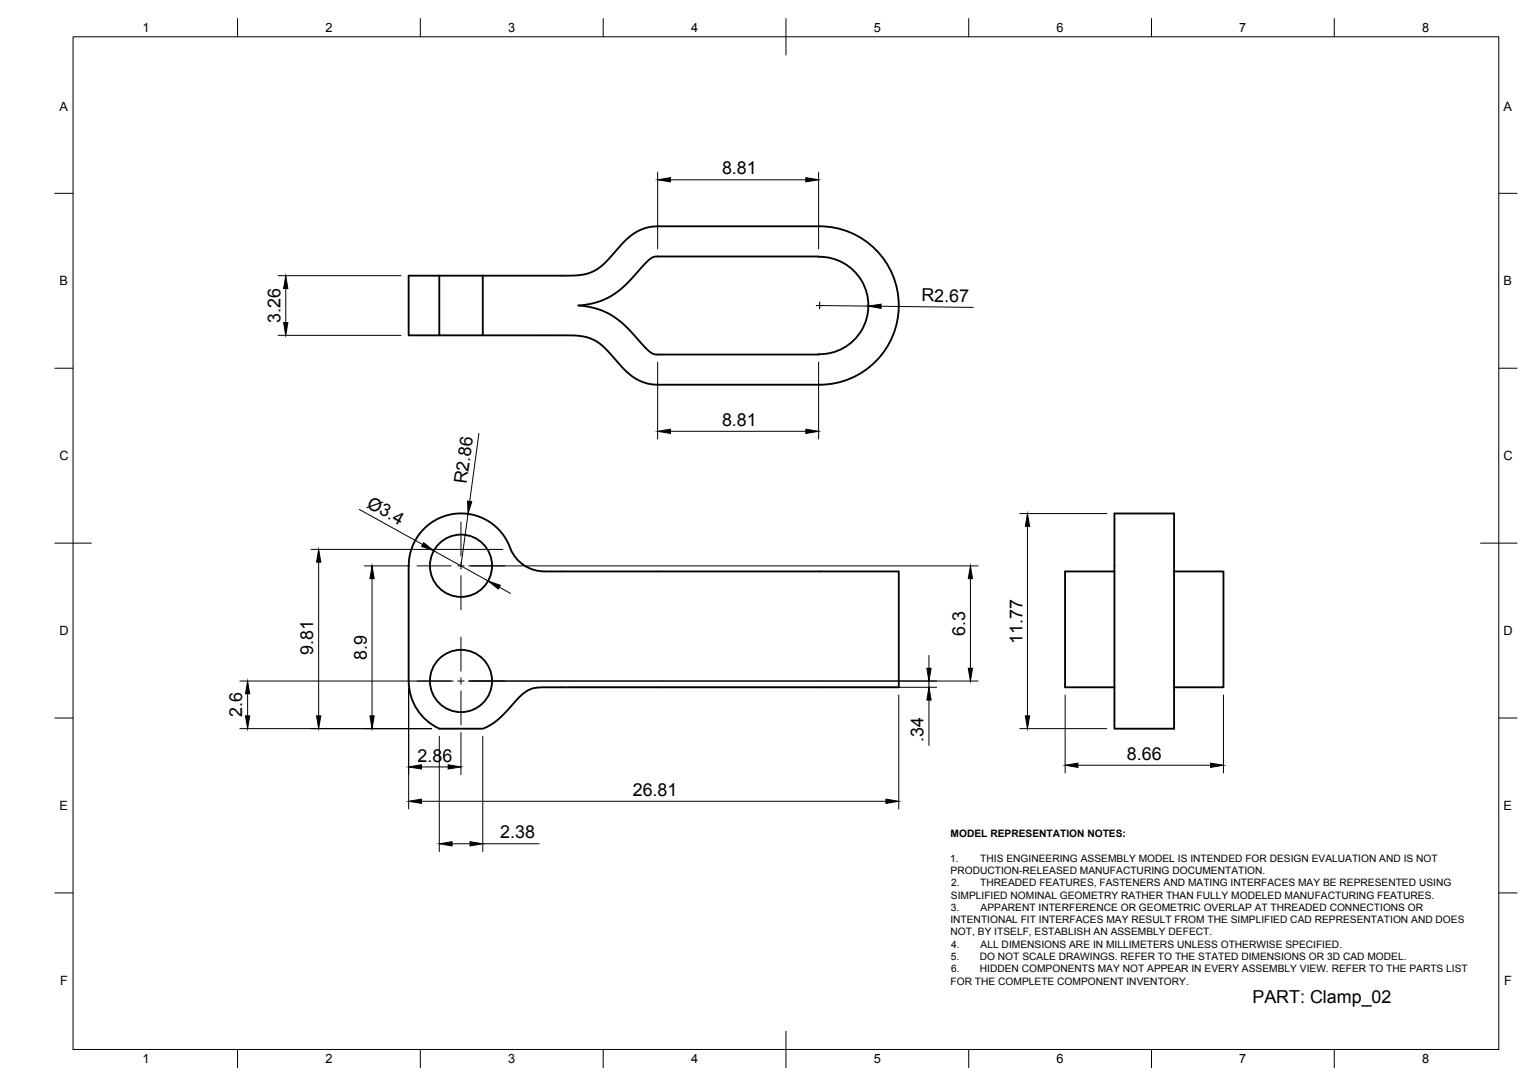
ISO-10303-21;
HEADER;
/* Generated by software containing ST-Developer
 * from STEP Tools, Inc. (www.steptools.com) 
 */

FILE_DESCRIPTION(
/* description */ (''),
/* implementation_level */ '2;1');

FILE_NAME(
/* name */ 'Clamp_02.step',
/* time_stamp */ '2026-10-05T16:20:14-07:00',
/* author */ (''),
/* organization */ (''),
/* preprocessor_version */ 'ST-DEVELOPER v20.2',
/* originating_system */ 'Autodesk Translation Framework v15.15.0.0',
/* authorisation */ '');

FILE_SCHEMA (('AUTOMOTIVE_DESIGN { 1 0 10303 214 3 1 1 }'));
ENDSEC;

DATA;
#10=MECHANICAL_DESIGN_GEOMETRIC_PRESENTATION_REPRESENTATION('',(#254),#23577);
#57=B_SPLINE_SURFACE_WITH_KNOTS('',5,1,((#22213,#22214),(#22215,#22216),
(#22217,#22218),(#22219,#22220),(#22221,#22222),(#22223,#22224),(#22225,
#22226),(#22227,#22228),(#22229,#22230),(#22231,#22232),(#22233,#22234),
(#22235,#22236),(#22237,#22238),(#22239,#22240),(#22241,#22242),(#22243,
#22244),(#22245,#22246),(#22247,#22248),(#22249,#22250),(#22251,#22252)),
 .UNSPECIFIED.,.F.,.F.,.F.,(6,1,1,1,1,1,1,1,1,1,1,1,1,1,1,6),(2,2),(0.,
0.0666666666666667,0.133333333333333,0.2,0.266666666666667,0.333333333333333,
0.4,0.466666666666667,0.533333333333333,0.6,0.666666666666667,0.733333333333333,
0.8,0.866666666666667,0.933333333333333,1.),(0.,1.44),.UNSPECIFIED.);
#58=B_SPLINE_SURFACE_WITH_KNOTS('',3,1,((#22299,#22300),(#22301,#22302),
(#22303,#22304),(#22305,#22306),(#22307,#22308),(#22309,#22310),(#22311,
#22312),(#22313,#22314),(#22315,#22316),(#22317,#22318),(#22319,#22320),
(#22321,#22322),(#22323,#22324),(#22325,#22326),(#22327,#22328),(#22329,
#22330)),.UNSPECIFIED.,.F.,.F.,.F.,(4,3,3,3,3,4),(2,2),(-1.,-0.857074929962035,
-0.680580226328136,-0.49099360586306,-0.247446976985656,0.),(0.,1.44229698166468),
 .UNSPECIFIED.);
#59=B_SPLINE_SURFACE_WITH_KNOTS('',3,1,((#22422,#22423),(#22424,#22425),
(#22426,#22427),(#22428,#22429),(#22430,#22431),(#22432,#22433),(#22434,
#22435),(#22436,#22437),(#22438,#22439),(#22440,#22441),(#22442,#22443),
(#22444,#22445),(#22446,#22447),(#22448,#22449),(#22450,#22451),(#22452,
#22453)),.UNSPECIFIED.,.F.,.F.,.F.,(4,3,3,3,3,4),(2,2),(-1.,-0.857074929962035,
-0.680580226328136,-0.49099360586306,-0.247446976985656,0.),(0.,1.44229698166468),
 .UNSPECIFIED.);
#60=B_SPLINE_SURFACE_WITH_KNOTS('',5,1,((#22519,#22520),(#22521,#22522),
(#22523,#22524),(#22525,#22526),(#22527,#22528),(#22529,#22530),(#22531,
#22532),(#22533,#22534),(#22535,#22536),(#22537,#22538),(#22539,#22540),
(#22541,#22542),(#22543,#22544),(#22545,#22546),(#22547,#22548),(#22549,
#22550),(#22551,#22552),(#22553,#22554),(#22555,#22556),(#22557,#22558)),
 .UNSPECIFIED.,.F.,.F.,.F.,(6,1,1,1,1,1,1,1,1,1,1,1,1,1,1,6),(2,2),(0.,
0.0666666666666667,0.133333333333333,0.2,0.266666666666667,0.333333333333333,
0.4,0.466666666666667,0.533333333333333,0.6,0.666666666666667,0.733333333333333,
0.8,0.866666666666667,0.933333333333333,1.),(0.,2.88),.UNSPECIFIED.);
#61=B_SPLINE_SURFACE_WITH_KNOTS('',5,1,((#22641,#22642),(#22643,#22644),
(#22645,#22646),(#22647,#22648),(#22649,#22650),(#22651,#22652),(#22653,
#22654),(#22655,#22656),(#22657,#22658),(#22659,#22660),(#22661,#22662),
(#22663,#22664),(#22665,#22666),(#22667,#22668),(#22669,#22670),(#22671,
#22672),(#22673,#22674),(#22675,#22676),(#22677,#22678),(#22679,#22680)),
 .UNSPECIFIED.,.F.,.F.,.F.,(6,1,1,1,1,1,1,1,1,1,1,1,1,1,1,6),(2,2),(0.,
0.0666666666666667,0.133333333333333,0.2,0.266666666666667,0.333333333333333,
0.4,0.466666666666667,0.533333333333333,0.6,0.666666666666667,0.733333333333333,
0.8,0.866666666666667,0.933333333333333,1.),(0.,1.44),.UNSPECIFIED.);
#181=B_SPLINE_CURVE_WITH_KNOTS('',5,(#22255,#22256,#22257,#22258,#22259,
#22260,#22261,#22262,#22263,#22264,#22265,#22266,#22267,#22268,#22269,#22270,
#22271,#22272,#22273,#22274),.UNSPECIFIED.,.F.,.F.,(6,1,1,1,1,1,1,1,1,1,
1,1,1,1,1,6),(0.,0.0666666666666667,0.133333333333333,0.2,0.266666666666667,
0.333333333333333,0.4,0.466666666666667,0.533333333333333,0.6,0.666666666666667,
0.733333333333333,0.8,0.866666666666667,0.933333333333333,1.),
 .UNSPECIFIED.);
#182=B_SPLINE_CURVE_WITH_KNOTS('',5,(#22278,#22279,#22280,#22281,#22282,
#22283,#22284,#22285,#22286,#22287,#22288,#22289,#22290,#22291,#22292,#22293,
#22294,#22295,#22296,#22297),.UNSPECIFIED.,.F.,.F.,(6,1,1,1,1,1,1,1,1,1,
1,1,1,1,1,6),(-1.,-0.933333333333333,-0.866666666666667,-0.8,-0.733333333333333,
-0.666666666666667,-0.6,-0.533333333333333,-0.466666666666667,-0.4,-0.333333333333333,
-0.266666666666667,-0.2,-0.133333333333333,-0.0666666666666667,0.),
 .UNSPECIFIED.);
#183=B_SPLINE_CURVE_WITH_KNOTS('',3,(#22335,#22336,#22337,#22338,#22339,
#22340,#22341,#22342,#22343,#22344,#22345,#22346,#22347,#22348,#22349,#22350),
 .UNSPECIFIED.,.F.,.F.,(4,3,3,3,3,4),(0.,0.247446976985656,0.49099360586306,
0.680580226328136,0.857074929962035,0.858875452739877),.UNSPECIFIED.);
#184=B_SPLINE_CURVE_WITH_KNOTS('',3,(#22353,#22354,#22355,#22356,#22357,
#22358,#22359,#22360,#22361,#22362,#22363,#22364),.UNSPECIFIED.,.F.,.F.,
(4,2,2,2,2,4),(-0.363889062449988,-0.363126279310584,-0.288348844096792,
-0.208024613752543,-0.10483855837836,0.),.UNSPECIFIED.);
#185=B_SPLINE_CURVE_WITH_KNOTS('',5,(#22372,#22373,#22374,#22375,#22376,
#22377,#22378,#22379,#22380,#22381,#22382,#22383,#22384,#22385,#22386,#22387,
#22388,#22389,#22390,#22391),.UNSPECIFIED.,.F.,.F.,(6,1,1,1,1,1,1,1,1,1,
1,1,1,1,1,6),(0.,0.0666666666666667,0.133333333333333,0.2,0.266666666666667,
0.333333333333333,0.4,0.466666666666667,0.533333333333333,0.6,0.666666666666667,
0.733333333333333,0.8,0.866666666666667,0.933333333333333,0.989745839682859),
 .UNSPECIFIED.);
#186=B_SPLINE_CURVE_WITH_KNOTS('',3,(#22455,#22456,#22457,#22458,#22459,
#22460,#22461,#22462,#22463,#22464,#22465,#22466),.UNSPECIFIED.,.F.,.F.,
(4,2,2,2,2,4),(-0.363889062449988,-0.363126279310585,-0.288348844096793,
-0.208024613752544,-0.10483855837836,0.),.UNSPECIFIED.);
#187=B_SPLINE_CURVE_WITH_KNOTS('',3,(#22469,#22470,#22471,#22472,#22473,
#22474,#22475,#22476,#22477,#22478,#22479,#22480,#22481,#22482,#22483,#22484),
 .UNSPECIFIED.,.F.,.F.,(4,3,3,3,3,4),(0.,0.247446976985656,0.49099360586306,
0.680580226328136,0.857074929962035,0.858875452739877),.UNSPECIFIED.);
#188=B_SPLINE_CURVE_WITH_KNOTS('',5,(#22491,#22492,#22493,#22494,#22495,
#22496,#22497,#22498,#22499,#22500,#22501,#22502,#22503,#22504,#22505,#22506,
#22507,#22508,#22509,#22510),.UNSPECIFIED.,.F.,.F.,(6,1,1,1,1,1,1,1,1,1,
1,1,1,1,1,6),(0.,0.0666666666666667,0.133333333333333,0.2,0.266666666666667,
0.333333333333333,0.4,0.466666666666667,0.533333333333333,0.6,0.666666666666667,
0.733333333333333,0.8,0.866666666666667,0.933333333333333,1.),
 .UNSPECIFIED.);
#189=B_SPLINE_CURVE_WITH_KNOTS('',5,(#22561,#22562,#22563,#22564,#22565,
#22566,#22567,#22568,#22569,#22570,#22571,#22572,#22573,#22574,#22575,#22576,
#22577,#22578,#22579,#22580),.UNSPECIFIED.,.F.,.F.,(6,1,1,1,1,1,1,1,1,1,
1,1,1,1,1,6),(0.,0.0666666666666667,0.133333333333333,0.2,0.266666666666667,
0.333333333333333,0.4,0.466666666666667,0.533333333333333,0.6,0.666666666666667,
0.733333333333333,0.8,0.866666666666667,0.933333333333333,0.989745839682859),
 .UNSPECIFIED.);
#190=B_SPLINE_CURVE_WITH_KNOTS('',5,(#22605,#22606,#22607,#22608,#22609,
#22610,#22611,#22612,#22613,#22614,#22615,#22616,#22617,#22618,#22619,#22620,
#22621,#22622,#22623,#22624),.UNSPECIFIED.,.F.,.F.,(6,1,1,1,1,1,1,1,1,1,
1,1,1,1,1,6),(-1.,-0.933333333333333,-0.866666666666667,-0.8,-0.733333333333333,
-0.666666666666667,-0.6,-0.533333333333333,-0.466666666666667,-0.4,-0.333333333333333,
-0.266666666666667,-0.2,-0.133333333333333,-0.0666666666666667,0.),
 .UNSPECIFIED.);
#236=SHAPE_REPRESENTATION_RELATIONSHIP('SRR','None',#23619,#245);
#245=ADVANCED_BREP_SHAPE_REPRESENTATION('',(#263),#23575);
#254=STYLED_ITEM('',(#23666),#263);
#263=MANIFOLD_SOLID_BREP('Body1',#4164);
#294=FACE_BOUND('',#822,.T.);
#295=FACE_BOUND('',#823,.T.);
#296=FACE_BOUND('',#829,.T.);
#297=FACE_BOUND('',#836,.T.);
#298=FACE_BOUND('',#842,.T.);
#299=FACE_BOUND('',#843,.T.);
#377=PLANE('',#4574);
#378=PLANE('',#4580);
#379=PLANE('',#4581);
#380=PLANE('',#4582);
#381=PLANE('',#4583);
#382=PLANE('',#4586);
#383=PLANE('',#4593);
#384=PLANE('',#4600);
#385=PLANE('',#4601);
#386=PLANE('',#4602);
#387=PLANE('',#4605);
#388=PLANE('',#4606);
#564=FACE_OUTER_BOUND('',#819,.T.);
#565=FACE_OUTER_BOUND('',#820,.T.);
#566=FACE_OUTER_BOUND('',#821,.T.);
#567=FACE_OUTER_BOUND('',#824,.T.);
#568=FACE_OUTER_BOUND('',#825,.T.);
#569=FACE_OUTER_BOUND('',#826,.T.);
#570=FACE_OUTER_BOUND('',#827,.T.);
#571=FACE_OUTER_BOUND('',#828,.T.);
#572=FACE_OUTER_BOUND('',#830,.T.);
#573=FACE_OUTER_BOUND('',#831,.T.);
#574=FACE_OUTER_BOUND('',#832,.T.);
#575=FACE_OUTER_BOUND('',#833,.T.);
#576=FACE_OUTER_BOUND('',#834,.T.);
#577=FACE_OUTER_BOUND('',#835,.T.);
#578=FACE_OUTER_BOUND('',#837,.T.);
#579=FACE_OUTER_BOUND('',#838,.T.);
#580=FACE_OUTER_BOUND('',#839,.T.);
#581=FACE_OUTER_BOUND('',#840,.T.);
#582=FACE_OUTER_BOUND('',#841,.T.);
#583=FACE_OUTER_BOUND('',#844,.T.);
#584=FACE_OUTER_BOUND('',#845,.T.);
#585=FACE_OUTER_BOUND('',#846,.T.);
#586=FACE_OUTER_BOUND('',#847,.T.);
#587=FACE_OUTER_BOUND('',#848,.T.);
#819=EDGE_LOOP('',(#3565,#3566,#3567,#3568));
#820=EDGE_LOOP('',(#3569,#3570,#3571,#3572));
#821=EDGE_LOOP('',(#3573,#3574,#3575,#3576,#3577,#3578,#3579,#3580,#3581));
#822=EDGE_LOOP('',(#3582));
#823=EDGE_LOOP('',(#3583));
#824=EDGE_LOOP('',(#3584,#3585,#3586,#3587));
#825=EDGE_LOOP('',(#3588,#3589,#3590,#3591));
#826=EDGE_LOOP('',(#3592,#3593,#3594,#3595));
#827=EDGE_LOOP('',(#3596,#3597,#3598,#3599));
#828=EDGE_LOOP('',(#3600,#3601,#3602,#3603,#3604,#3605,#3606,#3607));
#829=EDGE_LOOP('',(#3608,#3609,#3610,#3611,#3612,#3613,#3614));
#830=EDGE_LOOP('',(#3615,#3616,#3617,#3618));
#831=EDGE_LOOP('',(#3619,#3620,#3621,#3622));
#832=EDGE_LOOP('',(#3623,#3624,#3625,#3626));
#833=EDGE_LOOP('',(#3627,#3628,#3629,#3630));
#834=EDGE_LOOP('',(#3631,#3632,#3633,#3634));
#835=EDGE_LOOP('',(#3635,#3636,#3637,#3638,#3639,#3640,#3641,#3642));
#836=EDGE_LOOP('',(#3643,#3644,#3645,#3646,#3647,#3648,#3649));
#837=EDGE_LOOP('',(#3650,#3651,#3652,#3653));
#838=EDGE_LOOP('',(#3654,#3655,#3656,#3657));
#839=EDGE_LOOP('',(#3658,#3659,#3660,#3661));
#840=EDGE_LOOP('',(#3662,#3663,#3664,#3665));
#841=EDGE_LOOP('',(#3666,#3667,#3668,#3669,#3670,#3671,#3672,#3673,#3674));
#842=EDGE_LOOP('',(#3675));
#843=EDGE_LOOP('',(#3676));
#844=EDGE_LOOP('',(#3677,#3678,#3679,#3680));
#845=EDGE_LOOP('',(#3681,#3682,#3683,#3684));
#846=EDGE_LOOP('',(#3685,#3686,#3687,#3688));
#847=EDGE_LOOP('',(#3689,#3690,#3691,#3692));
#848=EDGE_LOOP('',(#3693,#3694,#3695,#3696));
#1102=LINE('',#22276,#1387);
#1103=LINE('',#22298,#1388);
#1104=LINE('',#22333,#1389);
#1105=LINE('',#22352,#1390);
#1106=LINE('',#22370,#1391);
#1107=LINE('',#22392,#1392);
#1108=LINE('',#22394,#1393);
#1109=LINE('',#22399,#1394);
#1110=LINE('',#22406,#1395);
#1111=LINE('',#22408,#1396);
#1112=LINE('',#22409,#1397);
#1113=LINE('',#22413,#1398);
#1114=LINE('',#22415,#1399);
#1115=LINE('',#22417,#1400);
#1116=LINE('',#22418,#1401);
#1117=LINE('',#22420,#1402);
#1118=LINE('',#22421,#1403);
#1119=LINE('',#22468,#1404);
#1120=LINE('',#22487,#1405);
#1121=LINE('',#22489,#1406);
#1122=LINE('',#22512,#1407);
#1123=LINE('',#22517,#1408);
#1124=LINE('',#22518,#1409);
#1125=LINE('',#22560,#1410);
#1126=LINE('',#22583,#1411);
#1127=LINE('',#22584,#1412);
#1128=LINE('',#22587,#1413);
#1129=LINE('',#22591,#1414);
#1130=LINE('',#22594,#1415);
#1131=LINE('',#22597,#1416);
#1132=LINE('',#22603,#1417);
#1133=LINE('',#22625,#1418);
#1134=LINE('',#22627,#1419);
#1135=LINE('',#22629,#1420);
#1136=LINE('',#22634,#1421);
#1137=LINE('',#22638,#1422);
#1138=LINE('',#22640,#1423);
#1139=LINE('',#22681,#1424);
#1140=LINE('',#22682,#1425);
#1141=LINE('',#22685,#1426);
#1142=LINE('',#22688,#1427);
#1143=LINE('',#22690,#1428);
#1387=VECTOR('',#5509,10.);
#1388=VECTOR('',#5510,10.);
#1389=VECTOR('',#5511,10.);
#1390=VECTOR('',#5512,10.);
#1391=VECTOR('',#5517,10.);
#1392=VECTOR('',#5518,10.);
#1393=VECTOR('',#5519,10.);
#1394=VECTOR('',#5524,10.);
#1395=VECTOR('',#5531,10.);
#1396=VECTOR('',#5532,10.);
#1397=VECTOR('',#5533,10.);
#1398=VECTOR('',#5536,10.);
#1399=VECTOR('',#5537,10.);
#1400=VECTOR('',#5538,10.);
#1401=VECTOR('',#5539,10.);
#1402=VECTOR('',#5542,10.);
#1403=VECTOR('',#5543,10.);
#1404=VECTOR('',#5544,10.);
#1405=VECTOR('',#5547,10.);
#1406=VECTOR('',#5548,10.);
#1407=VECTOR('',#5549,10.);
#1408=VECTOR('',#5554,10.);
#1409=VECTOR('',#5555,10.);
#1410=VECTOR('',#5556,10.);
#1411=VECTOR('',#5559,10.);
#1412=VECTOR('',#5560,10.);
#1413=VECTOR('',#5563,10.);
#1414=VECTOR('',#5568,10.);
#1415=VECTOR('',#5571,10.);
#1416=VECTOR('',#5574,10.);
#1417=VECTOR('',#5581,10.);
#1418=VECTOR('',#5582,10.);
#1419=VECTOR('',#5583,10.);
#1420=VECTOR('',#5584,10.);
#1421=VECTOR('',#5591,1.70133516896762);
#1422=VECTOR('',#5596,1.70133516896762);
#1423=VECTOR('',#5599,10.);
#1424=VECTOR('',#5600,10.);
#1425=VECTOR('',#5601,10.);
#1426=VECTOR('',#5606,10.);
#1427=VECTOR('',#5611,10.);
#1428=VECTOR('',#5614,10.);
#1584=CIRCLE('',#4575,2.8615696413584);
#1585=CIRCLE('',#4576,1.99589528357813);
#1586=CIRCLE('',#4577,2.8615696413584);
#1587=CIRCLE('',#4578,1.70133516896762);
#1588=CIRCLE('',#4579,1.70133516896762);
#1589=CIRCLE('',#4584,4.33051922028271);
#1590=CIRCLE('',#4585,2.66551922028271);
#1591=CIRCLE('',#4588,2.8615696413584);
#1592=CIRCLE('',#4590,2.8615696413584);
#1593=CIRCLE('',#4592,1.99589528357813);
#1594=CIRCLE('',#4594,4.33051922028271);
#1595=CIRCLE('',#4595,2.66551922028271);
#1596=CIRCLE('',#4597,1.70133516896762);
#1597=CIRCLE('',#4599,1.70133516896762);
#1951=VERTEX_POINT('',#22253);
#1952=VERTEX_POINT('',#22254);
#1953=VERTEX_POINT('',#22275);
#1954=VERTEX_POINT('',#22277);
#1955=VERTEX_POINT('',#22331);
#1956=VERTEX_POINT('',#22332);
#1957=VERTEX_POINT('',#22334);
#1958=VERTEX_POINT('',#22351);
#1959=VERTEX_POINT('',#22366);
#1960=VERTEX_POINT('',#22367);
#1961=VERTEX_POINT('',#22369);
#1962=VERTEX_POINT('',#22371);
#1963=VERTEX_POINT('',#22393);
#1964=VERTEX_POINT('',#22395);
#1965=VERTEX_POINT('',#22397);
#1966=VERTEX_POINT('',#22400);
#1967=VERTEX_POINT('',#22402);
#1968=VERTEX_POINT('',#22405);
#1969=VERTEX_POINT('',#22407);
#1970=VERTEX_POINT('',#22411);
#1971=VERTEX_POINT('',#22412);
#1972=VERTEX_POINT('',#22414);
#1973=VERTEX_POINT('',#22416);
#1974=VERTEX_POINT('',#22454);
#1975=VERTEX_POINT('',#22467);
#1976=VERTEX_POINT('',#22486);
#1977=VERTEX_POINT('',#22488);
#1978=VERTEX_POINT('',#22490);
#1979=VERTEX_POINT('',#22511);
#1980=VERTEX_POINT('',#22514);
#1981=VERTEX_POINT('',#22516);
#1982=VERTEX_POINT('',#22559);
#1983=VERTEX_POINT('',#22582);
#1984=VERTEX_POINT('',#22586);
#1985=VERTEX_POINT('',#22590);
#1986=VERTEX_POINT('',#22592);
#1987=VERTEX_POINT('',#22596);
#1988=VERTEX_POINT('',#22600);
#1989=VERTEX_POINT('',#22602);
#1990=VERTEX_POINT('',#22604);
#1991=VERTEX_POINT('',#22626);
#1992=VERTEX_POINT('',#22628);
#1993=VERTEX_POINT('',#22632);
#1994=VERTEX_POINT('',#22636);
#2499=EDGE_CURVE('',#1951,#1952,#181,.T.);
#2500=EDGE_CURVE('',#1951,#1953,#1102,.T.);
#2501=EDGE_CURVE('',#1954,#1953,#182,.T.);
#2502=EDGE_CURVE('',#1952,#1954,#1103,.T.);
#2503=EDGE_CURVE('',#1955,#1956,#1104,.T.);
#2504=EDGE_CURVE('',#1957,#1955,#183,.T.);
#2505=EDGE_CURVE('',#1957,#1958,#1105,.T.);
#2506=EDGE_CURVE('',#1956,#1958,#184,.T.);
#2507=EDGE_CURVE('',#1959,#1960,#1584,.T.);
#2508=EDGE_CURVE('',#1959,#1961,#1106,.T.);
#2509=EDGE_CURVE('',#1962,#1961,#185,.T.);
#2510=EDGE_CURVE('',#1952,#1962,#1107,.T.);
#2511=EDGE_CURVE('',#1963,#1954,#1108,.T.);
#2512=EDGE_CURVE('',#1964,#1963,#1585,.T.);
#2513=EDGE_CURVE('',#1965,#1964,#1586,.T.);
#2514=EDGE_CURVE('',#1960,#1965,#1109,.T.);
#2515=EDGE_CURVE('',#1966,#1966,#1587,.T.);
#2516=EDGE_CURVE('',#1967,#1967,#1588,.T.);
#2517=EDGE_CURVE('',#1968,#1951,#1110,.T.);
#2518=EDGE_CURVE('',#1968,#1969,#1111,.T.);
#2519=EDGE_CURVE('',#1953,#1969,#1112,.T.);
#2520=EDGE_CURVE('',#1970,#1971,#1113,.T.);
#2521=EDGE_CURVE('',#1970,#1972,#1114,.T.);
#2522=EDGE_CURVE('',#1973,#1972,#1115,.T.);
#2523=EDGE_CURVE('',#1971,#1973,#1116,.T.);
#2524=EDGE_CURVE('',#1958,#1970,#1117,.T.);
#2525=EDGE_CURVE('',#1972,#1957,#1118,.T.);
#2526=EDGE_CURVE('',#1956,#1974,#186,.T.);
#2527=EDGE_CURVE('',#1975,#1974,#1119,.T.);
#2528=EDGE_CURVE('',#1975,#1955,#187,.T.);
#2529=EDGE_CURVE('',#1962,#1976,#1120,.T.);
#2530=EDGE_CURVE('',#1977,#1976,#1121,.T.);
#2531=EDGE_CURVE('',#1978,#1977,#188,.T.);
#2532=EDGE_CURVE('',#1979,#1978,#1122,.T.);
#2533=EDGE_CURVE('',#1968,#1979,#1589,.T.);
#2534=EDGE_CURVE('',#1971,#1980,#1590,.T.);
#2535=EDGE_CURVE('',#1981,#1980,#1123,.T.);
#2536=EDGE_CURVE('',#1974,#1981,#1124,.T.);
#2537=EDGE_CURVE('',#1982,#1961,#1125,.T.);
#2538=EDGE_CURVE('',#1976,#1982,#189,.T.);
#2539=EDGE_CURVE('',#1959,#1983,#1126,.T.);
#2540=EDGE_CURVE('',#1983,#1982,#1127,.T.);
#2541=EDGE_CURVE('',#1984,#1960,#1128,.T.);
#2542=EDGE_CURVE('',#1983,#1984,#1591,.T.);
#2543=EDGE_CURVE('',#1964,#1985,#1129,.T.);
#2544=EDGE_CURVE('',#1986,#1985,#1592,.T.);
#2545=EDGE_CURVE('',#1965,#1986,#1130,.T.);
#2546=EDGE_CURVE('',#1963,#1987,#1131,.T.);
#2547=EDGE_CURVE('',#1985,#1987,#1593,.T.);
#2548=EDGE_CURVE('',#1988,#1969,#1594,.T.);
#2549=EDGE_CURVE('',#1989,#1988,#1132,.T.);
#2550=EDGE_CURVE('',#1990,#1989,#190,.T.);
#2551=EDGE_CURVE('',#1987,#1990,#1133,.T.);
#2552=EDGE_CURVE('',#1991,#1975,#1134,.T.);
#2553=EDGE_CURVE('',#1992,#1991,#1135,.T.);
#2554=EDGE_CURVE('',#1992,#1973,#1595,.T.);
#2555=EDGE_CURVE('',#1993,#1993,#1596,.T.);
#2556=EDGE_CURVE('',#1993,#1966,#1136,.T.);
#2557=EDGE_CURVE('',#1994,#1994,#1597,.T.);
#2558=EDGE_CURVE('',#1994,#1967,#1137,.T.);
#2559=EDGE_CURVE('',#1984,#1986,#1138,.T.);
#2560=EDGE_CURVE('',#1977,#1990,#1139,.T.);
#2561=EDGE_CURVE('',#1978,#1989,#1140,.T.);
#2562=EDGE_CURVE('',#1979,#1988,#1141,.T.);
#2563=EDGE_CURVE('',#1980,#1992,#1142,.T.);
#2564=EDGE_CURVE('',#1981,#1991,#1143,.T.);
#3565=ORIENTED_EDGE('',*,*,#2499,.F.);
#3566=ORIENTED_EDGE('',*,*,#2500,.T.);
#3567=ORIENTED_EDGE('',*,*,#2501,.F.);
#3568=ORIENTED_EDGE('',*,*,#2502,.F.);
#3569=ORIENTED_EDGE('',*,*,#2503,.F.);
#3570=ORIENTED_EDGE('',*,*,#2504,.F.);
#3571=ORIENTED_EDGE('',*,*,#2505,.T.);
#3572=ORIENTED_EDGE('',*,*,#2506,.F.);
#3573=ORIENTED_EDGE('',*,*,#2507,.F.);
#3574=ORIENTED_EDGE('',*,*,#2508,.T.);
#3575=ORIENTED_EDGE('',*,*,#2509,.F.);
#3576=ORIENTED_EDGE('',*,*,#2510,.F.);
#3577=ORIENTED_EDGE('',*,*,#2502,.T.);
#3578=ORIENTED_EDGE('',*,*,#2511,.F.);
#3579=ORIENTED_EDGE('',*,*,#2512,.F.);
#3580=ORIENTED_EDGE('',*,*,#2513,.F.);
#3581=ORIENTED_EDGE('',*,*,#2514,.F.);
#3582=ORIENTED_EDGE('',*,*,#2515,.F.);
#3583=ORIENTED_EDGE('',*,*,#2516,.F.);
#3584=ORIENTED_EDGE('',*,*,#2517,.F.);
#3585=ORIENTED_EDGE('',*,*,#2518,.T.);
#3586=ORIENTED_EDGE('',*,*,#2519,.F.);
#3587=ORIENTED_EDGE('',*,*,#2500,.F.);
#3588=ORIENTED_EDGE('',*,*,#2520,.F.);
#3589=ORIENTED_EDGE('',*,*,#2521,.T.);
#3590=ORIENTED_EDGE('',*,*,#2522,.F.);
#3591=ORIENTED_EDGE('',*,*,#2523,.F.);
#3592=ORIENTED_EDGE('',*,*,#2524,.F.);
#3593=ORIENTED_EDGE('',*,*,#2505,.F.);
#3594=ORIENTED_EDGE('',*,*,#2525,.F.);
#3595=ORIENTED_EDGE('',*,*,#2521,.F.);
#3596=ORIENTED_EDGE('',*,*,#2503,.T.);
#3597=ORIENTED_EDGE('',*,*,#2526,.T.);
#3598=ORIENTED_EDGE('',*,*,#2527,.F.);
#3599=ORIENTED_EDGE('',*,*,#2528,.T.);
#3600=ORIENTED_EDGE('',*,*,#2529,.T.);
#3601=ORIENTED_EDGE('',*,*,#2530,.F.);
#3602=ORIENTED_EDGE('',*,*,#2531,.F.);
#3603=ORIENTED_EDGE('',*,*,#2532,.F.);
#3604=ORIENTED_EDGE('',*,*,#2533,.F.);
#3605=ORIENTED_EDGE('',*,*,#2517,.T.);
#3606=ORIENTED_EDGE('',*,*,#2499,.T.);
#3607=ORIENTED_EDGE('',*,*,#2510,.T.);
#3608=ORIENTED_EDGE('',*,*,#2506,.T.);
#3609=ORIENTED_EDGE('',*,*,#2524,.T.);
#3610=ORIENTED_EDGE('',*,*,#2520,.T.);
#3611=ORIENTED_EDGE('',*,*,#2534,.T.);
#3612=ORIENTED_EDGE('',*,*,#2535,.F.);
#3613=ORIENTED_EDGE('',*,*,#2536,.F.);
#3614=ORIENTED_EDGE('',*,*,#2526,.F.);
#3615=ORIENTED_EDGE('',*,*,#2537,.F.);
#3616=ORIENTED_EDGE('',*,*,#2538,.F.);
#3617=ORIENTED_EDGE('',*,*,#2529,.F.);
#3618=ORIENTED_EDGE('',*,*,#2509,.T.);
#3619=ORIENTED_EDGE('',*,*,#2539,.T.);
#3620=ORIENTED_EDGE('',*,*,#2540,.T.);
#3621=ORIENTED_EDGE('',*,*,#2537,.T.);
#3622=ORIENTED_EDGE('',*,*,#2508,.F.);
#3623=ORIENTED_EDGE('',*,*,#2541,.F.);
#3624=ORIENTED_EDGE('',*,*,#2542,.F.);
#3625=ORIENTED_EDGE('',*,*,#2539,.F.);
#3626=ORIENTED_EDGE('',*,*,#2507,.T.);
#3627=ORIENTED_EDGE('',*,*,#2543,.T.);
#3628=ORIENTED_EDGE('',*,*,#2544,.F.);
#3629=ORIENTED_EDGE('',*,*,#2545,.F.);
#3630=ORIENTED_EDGE('',*,*,#2513,.T.);
#3631=ORIENTED_EDGE('',*,*,#2546,.T.);
#3632=ORIENTED_EDGE('',*,*,#2547,.F.);
#3633=ORIENTED_EDGE('',*,*,#2543,.F.);
#3634=ORIENTED_EDGE('',*,*,#2512,.T.);
#3635=ORIENTED_EDGE('',*,*,#2546,.F.);
#3636=ORIENTED_EDGE('',*,*,#2511,.T.);
#3637=ORIENTED_EDGE('',*,*,#2501,.T.);
#3638=ORIENTED_EDGE('',*,*,#2519,.T.);
#3639=ORIENTED_EDGE('',*,*,#2548,.F.);
#3640=ORIENTED_EDGE('',*,*,#2549,.F.);
#3641=ORIENTED_EDGE('',*,*,#2550,.F.);
#3642=ORIENTED_EDGE('',*,*,#2551,.F.);
#3643=ORIENTED_EDGE('',*,*,#2528,.F.);
#3644=ORIENTED_EDGE('',*,*,#2552,.F.);
#3645=ORIENTED_EDGE('',*,*,#2553,.F.);
#3646=ORIENTED_EDGE('',*,*,#2554,.T.);
#3647=ORIENTED_EDGE('',*,*,#2522,.T.);
#3648=ORIENTED_EDGE('',*,*,#2525,.T.);
#3649=ORIENTED_EDGE('',*,*,#2504,.T.);
#3650=ORIENTED_EDGE('',*,*,#2555,.F.);
#3651=ORIENTED_EDGE('',*,*,#2556,.T.);
#3652=ORIENTED_EDGE('',*,*,#2515,.T.);
#3653=ORIENTED_EDGE('',*,*,#2556,.F.);
#3654=ORIENTED_EDGE('',*,*,#2557,.F.);
#3655=ORIENTED_EDGE('',*,*,#2558,.T.);
#3656=ORIENTED_EDGE('',*,*,#2516,.T.);
#3657=ORIENTED_EDGE('',*,*,#2558,.F.);
#3658=ORIENTED_EDGE('',*,*,#2545,.T.);
#3659=ORIENTED_EDGE('',*,*,#2559,.F.);
#3660=ORIENTED_EDGE('',*,*,#2541,.T.);
#3661=ORIENTED_EDGE('',*,*,#2514,.T.);
#3662=ORIENTED_EDGE('',*,*,#2531,.T.);
#3663=ORIENTED_EDGE('',*,*,#2560,.T.);
#3664=ORIENTED_EDGE('',*,*,#2550,.T.);
#3665=ORIENTED_EDGE('',*,*,#2561,.F.);
#3666=ORIENTED_EDGE('',*,*,#2542,.T.);
#3667=ORIENTED_EDGE('',*,*,#2559,.T.);
#3668=ORIENTED_EDGE('',*,*,#2544,.T.);
#3669=ORIENTED_EDGE('',*,*,#2547,.T.);
#3670=ORIENTED_EDGE('',*,*,#2551,.T.);
#3671=ORIENTED_EDGE('',*,*,#2560,.F.);
#3672=ORIENTED_EDGE('',*,*,#2530,.T.);
#3673=ORIENTED_EDGE('',*,*,#2538,.T.);
#3674=ORIENTED_EDGE('',*,*,#2540,.F.);
#3675=ORIENTED_EDGE('',*,*,#2555,.T.);
#3676=ORIENTED_EDGE('',*,*,#2557,.T.);
#3677=ORIENTED_EDGE('',*,*,#2532,.T.);
#3678=ORIENTED_EDGE('',*,*,#2561,.T.);
#3679=ORIENTED_EDGE('',*,*,#2549,.T.);
#3680=ORIENTED_EDGE('',*,*,#2562,.F.);
#3681=ORIENTED_EDGE('',*,*,#2533,.T.);
#3682=ORIENTED_EDGE('',*,*,#2562,.T.);
#3683=ORIENTED_EDGE('',*,*,#2548,.T.);
#3684=ORIENTED_EDGE('',*,*,#2518,.F.);
#3685=ORIENTED_EDGE('',*,*,#2534,.F.);
#3686=ORIENTED_EDGE('',*,*,#2523,.T.);
#3687=ORIENTED_EDGE('',*,*,#2554,.F.);
#3688=ORIENTED_EDGE('',*,*,#2563,.F.);
#3689=ORIENTED_EDGE('',*,*,#2535,.T.);
#3690=ORIENTED_EDGE('',*,*,#2563,.T.);
#3691=ORIENTED_EDGE('',*,*,#2553,.T.);
#3692=ORIENTED_EDGE('',*,*,#2564,.F.);
#3693=ORIENTED_EDGE('',*,*,#2536,.T.);
#3694=ORIENTED_EDGE('',*,*,#2564,.T.);
#3695=ORIENTED_EDGE('',*,*,#2552,.T.);
#3696=ORIENTED_EDGE('',*,*,#2527,.T.);
#3914=CYLINDRICAL_SURFACE('',#4587,2.8615696413584);
#3915=CYLINDRICAL_SURFACE('',#4589,2.8615696413584);
#3916=CYLINDRICAL_SURFACE('',#4591,1.99589528357813);
#3917=CYLINDRICAL_SURFACE('',#4596,1.70133516896762);
#3918=CYLINDRICAL_SURFACE('',#4598,1.70133516896762);
#3919=CYLINDRICAL_SURFACE('',#4603,4.33051922028271);
#3920=CYLINDRICAL_SURFACE('',#4604,2.66551922028271);
#4099=ADVANCED_FACE('',(#564),#57,.F.);
#4100=ADVANCED_FACE('',(#565),#58,.F.);
#4101=ADVANCED_FACE('',(#566,#294,#295),#377,.F.);
#4102=ADVANCED_FACE('',(#567),#378,.F.);
#4103=ADVANCED_FACE('',(#568),#379,.F.);
#4104=ADVANCED_FACE('',(#569),#380,.F.);
#4105=ADVANCED_FACE('',(#570),#59,.T.);
#4106=ADVANCED_FACE('',(#571,#296),#381,.F.);
#4107=ADVANCED_FACE('',(#572),#60,.F.);
#4108=ADVANCED_FACE('',(#573),#382,.F.);
#4109=ADVANCED_FACE('',(#574),#3914,.T.);
#4110=ADVANCED_FACE('',(#575),#3915,.T.);
#4111=ADVANCED_FACE('',(#576),#3916,.F.);
#4112=ADVANCED_FACE('',(#577,#297),#383,.F.);
#4113=ADVANCED_FACE('',(#578),#3917,.F.);
#4114=ADVANCED_FACE('',(#579),#3918,.F.);
#4115=ADVANCED_FACE('',(#580),#384,.T.);
#4116=ADVANCED_FACE('',(#581),#61,.T.);
#4117=ADVANCED_FACE('',(#582,#298,#299),#385,.T.);
#4118=ADVANCED_FACE('',(#583),#386,.T.);
#4119=ADVANCED_FACE('',(#584),#3919,.T.);
#4120=ADVANCED_FACE('',(#585),#3920,.F.);
#4121=ADVANCED_FACE('',(#586),#387,.T.);
#4122=ADVANCED_FACE('',(#587),#388,.T.);
#4164=CLOSED_SHELL('',(#4099,#4100,#4101,#4102,#4103,#4104,#4105,#4106,
#4107,#4108,#4109,#4110,#4111,#4112,#4113,#4114,#4115,#4116,#4117,#4118,
#4119,#4120,#4121,#4122));
#4573=AXIS2_PLACEMENT_3D('',#22212,#5507,#5508);
#4574=AXIS2_PLACEMENT_3D('',#22365,#5513,#5514);
#4575=AXIS2_PLACEMENT_3D('',#22368,#5515,#5516);
#4576=AXIS2_PLACEMENT_3D('',#22396,#5520,#5521);
#4577=AXIS2_PLACEMENT_3D('',#22398,#5522,#5523);
#4578=AXIS2_PLACEMENT_3D('',#22401,#5525,#5526);
#4579=AXIS2_PLACEMENT_3D('',#22403,#5527,#5528);
#4580=AXIS2_PLACEMENT_3D('',#22404,#5529,#5530);
#4581=AXIS2_PLACEMENT_3D('',#22410,#5534,#5535);
#4582=AXIS2_PLACEMENT_3D('',#22419,#5540,#5541);
#4583=AXIS2_PLACEMENT_3D('',#22485,#5545,#5546);
#4584=AXIS2_PLACEMENT_3D('',#22513,#5550,#5551);
#4585=AXIS2_PLACEMENT_3D('',#22515,#5552,#5553);
#4586=AXIS2_PLACEMENT_3D('',#22581,#5557,#5558);
#4587=AXIS2_PLACEMENT_3D('',#22585,#5561,#5562);
#4588=AXIS2_PLACEMENT_3D('',#22588,#5564,#5565);
#4589=AXIS2_PLACEMENT_3D('',#22589,#5566,#5567);
#4590=AXIS2_PLACEMENT_3D('',#22593,#5569,#5570);
#4591=AXIS2_PLACEMENT_3D('',#22595,#5572,#5573);
#4592=AXIS2_PLACEMENT_3D('',#22598,#5575,#5576);
#4593=AXIS2_PLACEMENT_3D('',#22599,#5577,#5578);
#4594=AXIS2_PLACEMENT_3D('',#22601,#5579,#5580);
#4595=AXIS2_PLACEMENT_3D('',#22630,#5585,#5586);
#4596=AXIS2_PLACEMENT_3D('',#22631,#5587,#5588);
#4597=AXIS2_PLACEMENT_3D('',#22633,#5589,#5590);
#4598=AXIS2_PLACEMENT_3D('',#22635,#5592,#5593);
#4599=AXIS2_PLACEMENT_3D('',#22637,#5594,#5595);
#4600=AXIS2_PLACEMENT_3D('',#22639,#5597,#5598);
#4601=AXIS2_PLACEMENT_3D('',#22683,#5602,#5603);
#4602=AXIS2_PLACEMENT_3D('',#22684,#5604,#5605);
#4603=AXIS2_PLACEMENT_3D('',#22686,#5607,#5608);
#4604=AXIS2_PLACEMENT_3D('',#22687,#5609,#5610);
#4605=AXIS2_PLACEMENT_3D('',#22689,#5612,#5613);
#4606=AXIS2_PLACEMENT_3D('',#22691,#5615,#5616);
#5507=DIRECTION('axis',(0.,0.,1.));
#5508=DIRECTION('refdir',(1.,0.,0.));
#5509=DIRECTION('',(0.,0.,1.));
#5510=DIRECTION('',(0.,0.,1.));
#5511=DIRECTION('',(0.,8.75964579554923E-17,-1.));
#5512=DIRECTION('',(0.,0.,-1.));
#5513=DIRECTION('center_axis',(0.,-1.,0.));
#5514=DIRECTION('ref_axis',(1.,0.,0.));
#5515=DIRECTION('center_axis',(0.,-1.,0.));
#5516=DIRECTION('ref_axis',(1.,0.,0.));
#5517=DIRECTION('',(-1.,0.,0.));
#5518=DIRECTION('',(1.,0.,0.));
#5519=DIRECTION('',(-1.,0.,0.));
#5520=DIRECTION('center_axis',(0.,1.,0.));
#5521=DIRECTION('ref_axis',(0.918783056912983,0.,-0.3947628330145));
#5522=DIRECTION('center_axis',(0.,-1.,0.));
#5523=DIRECTION('ref_axis',(1.,0.,0.));
#5524=DIRECTION('',(0.,0.,1.));
#5525=DIRECTION('center_axis',(0.,1.,0.));
#5526=DIRECTION('ref_axis',(1.,0.,0.));
#5527=DIRECTION('center_axis',(0.,1.,0.));
#5528=DIRECTION('ref_axis',(1.,0.,0.));
#5529=DIRECTION('center_axis',(0.,-1.,0.));
#5530=DIRECTION('ref_axis',(1.,0.,0.));
#5531=DIRECTION('',(1.,0.,0.));
#5532=DIRECTION('',(0.,0.,1.));
#5533=DIRECTION('',(-1.,0.,0.));
#5534=DIRECTION('center_axis',(-1.,0.,0.));
#5535=DIRECTION('ref_axis',(0.,-1.,0.));
#5536=DIRECTION('',(0.,-1.,0.));
#5537=DIRECTION('',(0.,0.,1.));
#5538=DIRECTION('',(0.,1.,0.));
#5539=DIRECTION('',(0.,0.,1.));
#5540=DIRECTION('center_axis',(0.,1.,0.));
#5541=DIRECTION('ref_axis',(-1.,0.,0.));
#5542=DIRECTION('',(-1.,0.,0.));
#5543=DIRECTION('',(1.,0.,0.));
#5544=DIRECTION('',(0.,0.,-1.));
#5545=DIRECTION('center_axis',(0.,0.,1.));
#5546=DIRECTION('ref_axis',(1.,0.,0.));
#5547=DIRECTION('',(0.,-1.,0.));
#5548=DIRECTION('',(1.,0.,0.));
#5549=DIRECTION('',(1.,0.,0.));
#5550=DIRECTION('center_axis',(0.,0.,1.));
#5551=DIRECTION('ref_axis',(1.,0.,0.));
#5552=DIRECTION('center_axis',(0.,0.,1.));
#5553=DIRECTION('ref_axis',(1.,0.,0.));
#5554=DIRECTION('',(0.,1.,0.));
#5555=DIRECTION('',(-1.,0.,0.));
#5556=DIRECTION('',(0.,1.,0.));
#5557=DIRECTION('center_axis',(0.,0.,1.));
#5558=DIRECTION('ref_axis',(1.,0.,0.));
#5559=DIRECTION('',(0.,-1.,0.));
#5560=DIRECTION('',(-1.,0.,0.));
#5561=DIRECTION('center_axis',(0.,1.,0.));
#5562=DIRECTION('ref_axis',(1.,0.,0.));
#5563=DIRECTION('',(0.,1.,0.));
#5564=DIRECTION('center_axis',(0.,-1.,0.));
#5565=DIRECTION('ref_axis',(1.,0.,0.));
#5566=DIRECTION('center_axis',(0.,1.,0.));
#5567=DIRECTION('ref_axis',(1.,0.,0.));
#5568=DIRECTION('',(0.,-1.,0.));
#5569=DIRECTION('center_axis',(0.,-1.,0.));
#5570=DIRECTION('ref_axis',(1.,0.,0.));
#5571=DIRECTION('',(0.,-1.,0.));
#5572=DIRECTION('center_axis',(0.,1.,0.));
#5573=DIRECTION('ref_axis',(0.918783056912983,0.,-0.3947628330145));
#5574=DIRECTION('',(0.,-1.,0.));
#5575=DIRECTION('center_axis',(0.,1.,0.));
#5576=DIRECTION('ref_axis',(0.918783056912983,0.,-0.3947628330145));
#5577=DIRECTION('center_axis',(0.,0.,-1.));
#5578=DIRECTION('ref_axis',(-1.,0.,0.));
#5579=DIRECTION('center_axis',(0.,0.,-1.));
#5580=DIRECTION('ref_axis',(1.,0.,0.));
#5581=DIRECTION('',(-1.,0.,0.));
#5582=DIRECTION('',(-1.,0.,0.));
#5583=DIRECTION('',(1.,0.,0.));
#5584=DIRECTION('',(0.,-1.,0.));
#5585=DIRECTION('center_axis',(0.,0.,-1.));
#5586=DIRECTION('ref_axis',(1.,0.,0.));
#5587=DIRECTION('center_axis',(0.,1.,0.));
#5588=DIRECTION('ref_axis',(1.,0.,0.));
#5589=DIRECTION('center_axis',(0.,1.,0.));
#5590=DIRECTION('ref_axis',(1.,0.,0.));
#5591=DIRECTION('',(0.,1.,0.));
#5592=DIRECTION('center_axis',(0.,1.,0.));
#5593=DIRECTION('ref_axis',(1.,0.,0.));
#5594=DIRECTION('center_axis',(0.,1.,0.));
#5595=DIRECTION('ref_axis',(1.,0.,0.));
#5596=DIRECTION('',(0.,1.,0.));
#5597=DIRECTION('center_axis',(1.,0.,0.));
#5598=DIRECTION('ref_axis',(0.,1.,0.));
#5599=DIRECTION('',(0.,0.,1.));
#5600=DIRECTION('',(0.,0.,1.));
#5601=DIRECTION('',(0.,0.,1.));
#5602=DIRECTION('center_axis',(0.,-1.,0.));
#5603=DIRECTION('ref_axis',(1.,0.,0.));
#5604=DIRECTION('center_axis',(0.,-1.,0.));
#5605=DIRECTION('ref_axis',(1.,0.,0.));
#5606=DIRECTION('',(0.,0.,1.));
#5607=DIRECTION('center_axis',(0.,0.,1.));
#5608=DIRECTION('ref_axis',(-1.,1.22464679914735E-16,0.));
#5609=DIRECTION('center_axis',(0.,0.,1.));
#5610=DIRECTION('ref_axis',(-1.,1.22464679914735E-16,0.));
#5611=DIRECTION('',(0.,0.,1.));
#5612=DIRECTION('center_axis',(1.,0.,0.));
#5613=DIRECTION('ref_axis',(0.,1.,0.));
#5614=DIRECTION('',(0.,0.,1.));
#5615=DIRECTION('center_axis',(0.,1.,0.));
#5616=DIRECTION('ref_axis',(-1.,0.,0.));
#22212=CARTESIAN_POINT('',(0.,0.,0.));
#22213=CARTESIAN_POINT('Ctrl Pts',(13.9521549326808,4.33051922028271,-3.));
#22214=CARTESIAN_POINT('Ctrl Pts',(13.9521549326808,4.33051922028271,11.4));
#22215=CARTESIAN_POINT('Ctrl Pts',(14.0367700658778,4.33051922028271,-3.));
#22216=CARTESIAN_POINT('Ctrl Pts',(14.0367700658778,4.33051922028271,11.4));
#22217=CARTESIAN_POINT('Ctrl Pts',(14.2036369078635,4.3237071977066,-3.));
#22218=CARTESIAN_POINT('Ctrl Pts',(14.2036369078635,4.3237071977066,11.4));
#22219=CARTESIAN_POINT('Ctrl Pts',(14.4468469322399,4.29305314840303,-3.));
#22220=CARTESIAN_POINT('Ctrl Pts',(14.4468469322399,4.29305314840303,11.4));
#22221=CARTESIAN_POINT('Ctrl Pts',(14.7569409494257,4.21100033264776,-3.));
#22222=CARTESIAN_POINT('Ctrl Pts',(14.7569409494257,4.21100033264776,11.4));
#22223=CARTESIAN_POINT('Ctrl Pts',(15.1212896693278,4.03949049111154,-3.));
#22224=CARTESIAN_POINT('Ctrl Pts',(15.1212896693278,4.03949049111154,11.4));
#22225=CARTESIAN_POINT('Ctrl Pts',(15.4636185066764,3.80138932605477,-3.));
#22226=CARTESIAN_POINT('Ctrl Pts',(15.4636185066764,3.80138932605477,11.4));
#22227=CARTESIAN_POINT('Ctrl Pts',(15.7866049591328,3.50410652905647,-3.));
#22228=CARTESIAN_POINT('Ctrl Pts',(15.7866049591328,3.50410652905647,11.4));
#22229=CARTESIAN_POINT('Ctrl Pts',(16.0950135392462,3.16285055044176,-3.));
#22230=CARTESIAN_POINT('Ctrl Pts',(16.0950135392462,3.16285055044176,11.4));
#22231=CARTESIAN_POINT('Ctrl Pts',(16.396392567999,2.80347808583323,-3.));
#22232=CARTESIAN_POINT('Ctrl Pts',(16.396392567999,2.80347808583323,11.4));
#22233=CARTESIAN_POINT('Ctrl Pts',(16.6994685020962,2.45665970286042,-3.));
#22234=CARTESIAN_POINT('Ctrl Pts',(16.6994685020962,2.45665970286042,11.4));
#22235=CARTESIAN_POINT('Ctrl Pts',(17.0126841408516,2.15256650575318,-3.));
#22236=CARTESIAN_POINT('Ctrl Pts',(17.0126841408516,2.15256650575318,11.4));
#22237=CARTESIAN_POINT('Ctrl Pts',(17.3426063821155,1.91508101584403,-3.));
#22238=CARTESIAN_POINT('Ctrl Pts',(17.3426063821155,1.91508101584403,11.4));
#22239=CARTESIAN_POINT('Ctrl Pts',(17.6925082784732,1.75662630260534,-3.));
#22240=CARTESIAN_POINT('Ctrl Pts',(17.6925082784732,1.75662630260534,11.4));
#22241=CARTESIAN_POINT('Ctrl Pts',(18.0602469444161,1.6704655276535,-3.));
#22242=CARTESIAN_POINT('Ctrl Pts',(18.0602469444161,1.6704655276535,11.4));
#22243=CARTESIAN_POINT('Ctrl Pts',(18.4399535686149,1.63662374391445,-3.));
#22244=CARTESIAN_POINT('Ctrl Pts',(18.4399535686149,1.63662374391445,11.4));
#22245=CARTESIAN_POINT('Ctrl Pts',(18.7476534820197,1.63200385678456,-3.));
#22246=CARTESIAN_POINT('Ctrl Pts',(18.7476534820197,1.63200385678456,11.4));
#22247=CARTESIAN_POINT('Ctrl Pts',(18.9779068684107,1.63172180635354,-3.));
#22248=CARTESIAN_POINT('Ctrl Pts',(18.9779068684107,1.63172180635354,11.4));
#22249=CARTESIAN_POINT('Ctrl Pts',(19.1308048362197,1.63165946910082,-3.));
#22250=CARTESIAN_POINT('Ctrl Pts',(19.1308048362197,1.63165946910082,11.4));
#22251=CARTESIAN_POINT('Ctrl Pts',(19.2071026744088,1.63165946910082,-3.));
#22252=CARTESIAN_POINT('Ctrl Pts',(19.2071026744088,1.63165946910082,11.4));
#22253=CARTESIAN_POINT('',(13.9521549326808,4.33051922028271,-0.737782898536615));
#22254=CARTESIAN_POINT('',(19.2071026744088,1.63165946910082,-0.737782898536615));
#22255=CARTESIAN_POINT('Ctrl Pts',(13.9521549326808,4.33051922028271,-0.737782898536615));
#22256=CARTESIAN_POINT('Ctrl Pts',(14.0367700658778,4.33051922028271,-0.737782898536615));
#22257=CARTESIAN_POINT('Ctrl Pts',(14.2036369078635,4.3237071977066,-0.737782898536615));
#22258=CARTESIAN_POINT('Ctrl Pts',(14.4468469322399,4.29305314840303,-0.737782898536615));
#22259=CARTESIAN_POINT('Ctrl Pts',(14.7569409494257,4.21100033264776,-0.737782898536615));
#22260=CARTESIAN_POINT('Ctrl Pts',(15.1212896693278,4.03949049111154,-0.737782898536615));
#22261=CARTESIAN_POINT('Ctrl Pts',(15.4636185066764,3.80138932605477,-0.737782898536615));
#22262=CARTESIAN_POINT('Ctrl Pts',(15.7866049591328,3.50410652905647,-0.737782898536615));
#22263=CARTESIAN_POINT('Ctrl Pts',(16.0950135392462,3.16285055044176,-0.737782898536615));
#22264=CARTESIAN_POINT('Ctrl Pts',(16.396392567999,2.80347808583323,-0.737782898536615));
#22265=CARTESIAN_POINT('Ctrl Pts',(16.6994685020962,2.45665970286042,-0.737782898536615));
#22266=CARTESIAN_POINT('Ctrl Pts',(17.0126841408516,2.15256650575318,-0.737782898536615));
#22267=CARTESIAN_POINT('Ctrl Pts',(17.3426063821155,1.91508101584403,-0.737782898536615));
#22268=CARTESIAN_POINT('Ctrl Pts',(17.6925082784732,1.75662630260534,-0.737782898536615));
#22269=CARTESIAN_POINT('Ctrl Pts',(18.0602469444161,1.6704655276535,-0.737782898536615));
#22270=CARTESIAN_POINT('Ctrl Pts',(18.4399535686149,1.63662374391445,-0.737782898536615));
#22271=CARTESIAN_POINT('Ctrl Pts',(18.7476534820197,1.63200385678456,-0.737782898536615));
#22272=CARTESIAN_POINT('Ctrl Pts',(18.9779068684107,1.63172180635354,-0.737782898536615));
#22273=CARTESIAN_POINT('Ctrl Pts',(19.1308048362197,1.63165946910082,-0.737782898536615));
#22274=CARTESIAN_POINT('Ctrl Pts',(19.2071026744088,1.63165946910082,-0.737782898536615));
#22275=CARTESIAN_POINT('',(13.9521549326808,4.33051922028271,5.59936274946018));
#22276=CARTESIAN_POINT('',(13.9521549326808,4.33051922028271,0.));
#22277=CARTESIAN_POINT('',(19.2071026744088,1.63165946910082,5.59936274946018));
#22278=CARTESIAN_POINT('Ctrl Pts',(19.2071026744088,1.63165946910082,5.59936274946018));
#22279=CARTESIAN_POINT('Ctrl Pts',(19.1308048362197,1.63165946910082,5.59936274946018));
#22280=CARTESIAN_POINT('Ctrl Pts',(18.9779068684107,1.63172180635354,5.59936274946018));
#22281=CARTESIAN_POINT('Ctrl Pts',(18.7476534820197,1.63200385678456,5.59936274946018));
#22282=CARTESIAN_POINT('Ctrl Pts',(18.4399535686149,1.63662374391445,5.59936274946018));
#22283=CARTESIAN_POINT('Ctrl Pts',(18.0602469444161,1.6704655276535,5.59936274946018));
#22284=CARTESIAN_POINT('Ctrl Pts',(17.6925082784732,1.75662630260534,5.59936274946018));
#22285=CARTESIAN_POINT('Ctrl Pts',(17.3426063821155,1.91508101584403,5.59936274946018));
#22286=CARTESIAN_POINT('Ctrl Pts',(17.0126841408516,2.15256650575318,5.59936274946018));
#22287=CARTESIAN_POINT('Ctrl Pts',(16.6994685020962,2.45665970286042,5.59936274946018));
#22288=CARTESIAN_POINT('Ctrl Pts',(16.396392567999,2.80347808583323,5.59936274946018));
#22289=CARTESIAN_POINT('Ctrl Pts',(16.0950135392462,3.16285055044176,5.59936274946018));
#22290=CARTESIAN_POINT('Ctrl Pts',(15.7866049591328,3.50410652905647,5.59936274946018));
#22291=CARTESIAN_POINT('Ctrl Pts',(15.4636185066764,3.80138932605477,5.59936274946018));
#22292=CARTESIAN_POINT('Ctrl Pts',(15.1212896693278,4.03949049111154,5.59936274946018));
#22293=CARTESIAN_POINT('Ctrl Pts',(14.7569409494257,4.21100033264776,5.59936274946018));
#22294=CARTESIAN_POINT('Ctrl Pts',(14.4468469322399,4.29305314840303,5.59936274946018));
#22295=CARTESIAN_POINT('Ctrl Pts',(14.2036369078635,4.3237071977066,5.59936274946018));
#22296=CARTESIAN_POINT('Ctrl Pts',(14.0367700658778,4.33051922028271,5.59936274946018));
#22297=CARTESIAN_POINT('Ctrl Pts',(13.9521549326808,4.33051922028271,5.59936274946018));
#22298=CARTESIAN_POINT('',(19.2071026744088,1.63165946910082,0.));
#22299=CARTESIAN_POINT('Ctrl Pts',(19.2071026744088,-0.0183405308991755,
-3.01914151387231));
#22300=CARTESIAN_POINT('Ctrl Pts',(19.2071026744088,-0.0183405308991755,
11.4038283027745));
#22301=CARTESIAN_POINT('Ctrl Pts',(18.932554067018,-0.0183405308991755,
-3.01914151387231));
#22302=CARTESIAN_POINT('Ctrl Pts',(18.932554067018,-0.0183405308991755,
11.4038283027745));
#22303=CARTESIAN_POINT('Ctrl Pts',(18.6452346172082,-0.0244648993437209,
-3.01914151387231));
#22304=CARTESIAN_POINT('Ctrl Pts',(18.6452346172082,-0.0244648993437209,
11.4038283027745));
#22305=CARTESIAN_POINT('Ctrl Pts',(18.2737554003772,0.00094178007888357,
-3.01914151387231));
#22306=CARTESIAN_POINT('Ctrl Pts',(18.2737554003772,0.00094178007888357,
11.4038283027745));
#22307=CARTESIAN_POINT('Ctrl Pts',(17.815024722384,0.0323158724884442,-3.01914151387231));
#22308=CARTESIAN_POINT('Ctrl Pts',(17.815024722384,0.0323158724884442,11.4038283027745));
#22309=CARTESIAN_POINT('Ctrl Pts',(17.2029954141084,0.14276585350144,-3.01914151387231));
#22310=CARTESIAN_POINT('Ctrl Pts',(17.2029954141084,0.14276585350144,11.4038283027745));
#22311=CARTESIAN_POINT('Ctrl Pts',(16.6476240631459,0.436436950410268,-3.01914151387231));
#22312=CARTESIAN_POINT('Ctrl Pts',(16.6476240631459,0.436436950410268,11.4038283027745));
#22313=CARTESIAN_POINT('Ctrl Pts',(16.0510567137341,0.751891803416538,-3.01914151387231));
#22314=CARTESIAN_POINT('Ctrl Pts',(16.0510567137341,0.751891803416538,11.4038283027745));
#22315=CARTESIAN_POINT('Ctrl Pts',(15.6027736445726,1.21202503656501,-3.01914151387231));
#22316=CARTESIAN_POINT('Ctrl Pts',(15.6027736445726,1.21202503656501,11.4038283027745));
#22317=CARTESIAN_POINT('Ctrl Pts',(15.2713584598603,1.58690028117533,-3.01914151387231));
#22318=CARTESIAN_POINT('Ctrl Pts',(15.2713584598603,1.58690028117533,11.4038283027745));
#22319=CARTESIAN_POINT('Ctrl Pts',(14.8456161221497,2.0684722499697,-3.01914151387231));
#22320=CARTESIAN_POINT('Ctrl Pts',(14.8456161221497,2.0684722499697,11.4038283027745));
#22321=CARTESIAN_POINT('Ctrl Pts',(14.5613685394243,2.40143629916816,-3.01914151387231));
#22322=CARTESIAN_POINT('Ctrl Pts',(14.5613685394243,2.40143629916816,11.4038283027745));
#22323=CARTESIAN_POINT('Ctrl Pts',(14.3828812435025,2.53302458721095,-3.01914151387231));
#22324=CARTESIAN_POINT('Ctrl Pts',(14.3828812435025,2.53302458721095,11.4038283027745));
#22325=CARTESIAN_POINT('Ctrl Pts',(14.201535511025,2.66672023404866,-3.01914151387231));
#22326=CARTESIAN_POINT('Ctrl Pts',(14.201535511025,2.66672023404866,11.4038283027745));
#22327=CARTESIAN_POINT('Ctrl Pts',(14.14690312219,2.68051922028271,-3.01914151387231));
#22328=CARTESIAN_POINT('Ctrl Pts',(14.14690312219,2.68051922028271,11.4038283027745));
#22329=CARTESIAN_POINT('Ctrl Pts',(13.9521549326808,2.68051922028271,-3.01914151387231));
#22330=CARTESIAN_POINT('Ctrl Pts',(13.9521549326808,2.68051922028271,11.4038283027745));
#22331=CARTESIAN_POINT('',(18.2877550231844,1.59204426907891E-25,5.59936274946018));
#22332=CARTESIAN_POINT('',(18.2877550231844,-7.96022134539453E-26,-0.737782898536615));
#22333=CARTESIAN_POINT('',(18.2877582116991,5.55111512312578E-16,5.59936274946018));
#22334=CARTESIAN_POINT('',(13.9521549326808,2.68051922028271,5.59936274946018));
#22335=CARTESIAN_POINT('Ctrl Pts',(13.9521549326808,2.68051922028271,5.59936274946018));
#22336=CARTESIAN_POINT('Ctrl Pts',(14.14690312219,2.68051922028271,5.59936274946018));
#22337=CARTESIAN_POINT('Ctrl Pts',(14.201535511025,2.66672023404866,5.59936274946018));
#22338=CARTESIAN_POINT('Ctrl Pts',(14.3828812435025,2.53302458721095,5.59936274946018));
#22339=CARTESIAN_POINT('Ctrl Pts',(14.5613685394243,2.40143629916816,5.59936274946018));
#22340=CARTESIAN_POINT('Ctrl Pts',(14.8456161221497,2.0684722499697,5.59936274946018));
#22341=CARTESIAN_POINT('Ctrl Pts',(15.2713584598603,1.58690028117533,5.59936274946018));
#22342=CARTESIAN_POINT('Ctrl Pts',(15.6027736445726,1.21202503656501,5.59936274946018));
#22343=CARTESIAN_POINT('Ctrl Pts',(16.0510567137341,0.751891803416538,5.59936274946018));
#22344=CARTESIAN_POINT('Ctrl Pts',(16.6476240631459,0.436436950410268,5.59936274946018));
#22345=CARTESIAN_POINT('Ctrl Pts',(17.2029954141084,0.14276585350144,5.59936274946018));
#22346=CARTESIAN_POINT('Ctrl Pts',(17.815024722384,0.0323158724884442,5.59936274946018));
#22347=CARTESIAN_POINT('Ctrl Pts',(18.2737554003772,0.00094178007888357,
5.59936274946018));
#22348=CARTESIAN_POINT('Ctrl Pts',(18.2784351727308,0.000621715131582291,
5.59936274946018));
#22349=CARTESIAN_POINT('Ctrl Pts',(18.2831015888222,0.000306654201738636,
5.59936274946018));
#22350=CARTESIAN_POINT('Ctrl Pts',(18.2877547913768,-3.47799384755541E-6,
5.59936274946018));
#22351=CARTESIAN_POINT('',(13.9521549326808,2.68051922028271,-0.737782898536615));
#22352=CARTESIAN_POINT('',(13.9521549326808,2.68051922028271,0.));
#22353=CARTESIAN_POINT('Ctrl Pts',(18.2877536206758,-3.39996748941005E-6,
-0.737782898536615));
#22354=CARTESIAN_POINT('Ctrl Pts',(18.2831008061387,0.000306707045957792,
-0.737782898536615));
#22355=CARTESIAN_POINT('Ctrl Pts',(18.278434780269,0.000621741973328407,
-0.737782898536615));
#22356=CARTESIAN_POINT('Ctrl Pts',(17.815024722384,0.0323158724884443,-0.737782898536615));
#22357=CARTESIAN_POINT('Ctrl Pts',(17.2029954141084,0.14276585350144,-0.737782898536615));
#22358=CARTESIAN_POINT('Ctrl Pts',(16.0510567137341,0.751891803416538,-0.737782898536615));
#22359=CARTESIAN_POINT('Ctrl Pts',(15.6027736445726,1.21202503656501,-0.737782898536615));
#22360=CARTESIAN_POINT('Ctrl Pts',(14.8456161221497,2.0684722499697,-0.737782898536615));
#22361=CARTESIAN_POINT('Ctrl Pts',(14.5613685394243,2.40143629916816,-0.737782898536615));
#22362=CARTESIAN_POINT('Ctrl Pts',(14.201535511025,2.66672023404866,-0.737782898536615));
#22363=CARTESIAN_POINT('Ctrl Pts',(14.14690312219,2.68051922028271,-0.737782898536615));
#22364=CARTESIAN_POINT('Ctrl Pts',(13.9521549326808,2.68051922028271,-0.737782898536615));
#22365=CARTESIAN_POINT('Origin',(19.2071026744088,1.63165946910082,0.));
#22366=CARTESIAN_POINT('',(25.8992960798277,1.63165946910082,-3.));
#22367=CARTESIAN_POINT('',(27.575916328613,1.63165946910082,-0.395297377936459));
#22368=CARTESIAN_POINT('Origin',(24.7143466872546,1.63165946910082,-0.395297377936459));
#22369=CARTESIAN_POINT('',(23.5207683417462,1.63165946910082,-3.));
#22370=CARTESIAN_POINT('',(19.2071026744088,1.63165946910082,-3.));
#22371=CARTESIAN_POINT('',(20.1650770882888,1.63165946910082,-0.737782898536615));
#22372=CARTESIAN_POINT('Ctrl Pts',(20.1650770882888,1.63165946910083,-0.737782898536615));
#22373=CARTESIAN_POINT('Ctrl Pts',(20.2051790492699,1.63165946910083,-0.737782898536615));
#22374=CARTESIAN_POINT('Ctrl Pts',(20.2856318058959,1.63165946910083,-0.738334262610078));
#22375=CARTESIAN_POINT('Ctrl Pts',(20.4070574409421,1.63165946910083,-0.740817279017836));
#22376=CARTESIAN_POINT('Ctrl Pts',(20.570466834294,1.63165946910083,-0.750031355028731));
#22377=CARTESIAN_POINT('Ctrl Pts',(20.7773607278973,1.63165946910083,-0.785302229564316));
#22378=CARTESIAN_POINT('Ctrl Pts',(20.9870805449298,1.63165946910083,-0.859882777793607));
#22379=CARTESIAN_POINT('Ctrl Pts',(21.1998878964781,1.63165946910083,-0.985918438087056));
#22380=CARTESIAN_POINT('Ctrl Pts',(21.4160984502468,1.63165946910083,-1.16513193018819));
#22381=CARTESIAN_POINT('Ctrl Pts',(21.6360629244597,1.63165946910083,-1.38851558520595));
#22382=CARTESIAN_POINT('Ctrl Pts',(21.8601428560791,1.63165946910083,-1.64103427806176));
#22383=CARTESIAN_POINT('Ctrl Pts',(22.0886743686473,1.63165946910083,-1.90460559759654));
#22384=CARTESIAN_POINT('Ctrl Pts',(22.3219273279567,1.63165946910083,-2.16140314464429));
#22385=CARTESIAN_POINT('Ctrl Pts',(22.5600378010161,1.63165946910083,-2.3973000769867));
#22386=CARTESIAN_POINT('Ctrl Pts',(22.8029682104327,1.63165946910083,-2.60422537589526));
#22387=CARTESIAN_POINT('Ctrl Pts',(23.0429827907474,1.63165946910083,-2.77271153031038));
#22388=CARTESIAN_POINT('Ctrl Pts',(23.2368431253681,1.63165946910083,-2.88095209536456));
#22389=CARTESIAN_POINT('Ctrl Pts',(23.3821028186482,1.63165946910083,-2.94712138325619));
#22390=CARTESIAN_POINT('Ctrl Pts',(23.4770787559704,1.63165946910083,-2.98421892689512));
#22391=CARTESIAN_POINT('Ctrl Pts',(23.5207683417462,1.63165946910083,-3.));
#22392=CARTESIAN_POINT('',(8.65639871597966,1.63165946910082,-0.737782898536615));
#22393=CARTESIAN_POINT('',(20.1650770882888,1.63165946910082,5.59936274946018));
#22394=CARTESIAN_POINT('',(19.6860898813488,1.63165946910082,5.59936274946018));
#22395=CARTESIAN_POINT('',(21.9988718582129,1.63165946910082,6.80735275649273));
#22396=CARTESIAN_POINT('Origin',(20.1650770882888,1.63165946910082,7.59525803303831));
#22397=CARTESIAN_POINT('',(27.575916328613,1.63165946910082,5.90470262206354));
#22398=CARTESIAN_POINT('Origin',(24.7143466872546,1.63165946910082,5.90470262206354));
#22399=CARTESIAN_POINT('',(27.575916328613,1.63165946910082,0.));
#22400=CARTESIAN_POINT('',(23.013011518287,1.63165946910082,5.90470262206354));
#22401=CARTESIAN_POINT('Origin',(24.7143466872546,1.63165946910082,5.90470262206354));
#22402=CARTESIAN_POINT('',(23.013011518287,1.63165946910082,-0.395297377936459));
#22403=CARTESIAN_POINT('Origin',(24.7143466872546,1.63165946910082,-0.395297377936459));
#22404=CARTESIAN_POINT('Origin',(5.09382715545311,4.33051922028271,0.));
#22405=CARTESIAN_POINT('',(5.09382715545311,4.33051922028271,-0.737782898536615));
#22406=CARTESIAN_POINT('',(1.59976095650181,4.33051922028271,-0.737782898536615));
#22407=CARTESIAN_POINT('',(5.09382715545311,4.33051922028271,5.59936274946018));
#22408=CARTESIAN_POINT('',(5.09382715545311,4.33051922028271,0.));
#22409=CARTESIAN_POINT('',(12.629452121871,4.33051922028271,5.59936274946018));
#22410=CARTESIAN_POINT('Origin',(5.1457717363639,2.68051922028271,0.));
#22411=CARTESIAN_POINT('',(5.1457717363639,2.68051922028271,-0.737782898536615));
#22412=CARTESIAN_POINT('',(5.1457717363639,2.6650130345292,-0.737782898536615));
#22413=CARTESIAN_POINT('',(5.1457717363639,1.34025961014136,-0.737782898536615));
#22414=CARTESIAN_POINT('',(5.1457717363639,2.68051922028271,5.59936274946018));
#22415=CARTESIAN_POINT('',(5.1457717363639,2.68051922028271,0.));
#22416=CARTESIAN_POINT('',(5.1457717363639,2.6650130345292,5.59936274946018));
#22417=CARTESIAN_POINT('',(5.1457717363639,1.34025961014136,5.59936274946018));
#22418=CARTESIAN_POINT('',(5.1457717363639,2.6650130345292,0.));
#22419=CARTESIAN_POINT('Origin',(13.9521549326808,2.68051922028271,0.));
#22420=CARTESIAN_POINT('',(6.02892484511565,2.68051922028271,-0.737782898536615));
#22421=CARTESIAN_POINT('',(17.0586160104848,2.68051922028271,5.59936274946018));
#22422=CARTESIAN_POINT('Ctrl Pts',(19.2071026744088,0.0183405308991755,
-3.01914151387231));
#22423=CARTESIAN_POINT('Ctrl Pts',(19.2071026744088,0.0183405308991755,
11.4038283027745));
#22424=CARTESIAN_POINT('Ctrl Pts',(18.932554067018,0.0183405308991755,-3.01914151387231));
#22425=CARTESIAN_POINT('Ctrl Pts',(18.932554067018,0.0183405308991755,11.4038283027745));
#22426=CARTESIAN_POINT('Ctrl Pts',(18.6452346172082,0.0244648993437209,
-3.01914151387231));
#22427=CARTESIAN_POINT('Ctrl Pts',(18.6452346172082,0.0244648993437209,
11.4038283027745));
#22428=CARTESIAN_POINT('Ctrl Pts',(18.2737554003772,-0.00094178007888357,
-3.01914151387231));
#22429=CARTESIAN_POINT('Ctrl Pts',(18.2737554003772,-0.00094178007888357,
11.4038283027745));
#22430=CARTESIAN_POINT('Ctrl Pts',(17.815024722384,-0.0323158724884442,
-3.01914151387231));
#22431=CARTESIAN_POINT('Ctrl Pts',(17.815024722384,-0.0323158724884442,
11.4038283027745));
#22432=CARTESIAN_POINT('Ctrl Pts',(17.2029954141084,-0.14276585350144,-3.01914151387231));
#22433=CARTESIAN_POINT('Ctrl Pts',(17.2029954141084,-0.14276585350144,11.4038283027745));
#22434=CARTESIAN_POINT('Ctrl Pts',(16.6476240631459,-0.436436950410268,
-3.01914151387231));
#22435=CARTESIAN_POINT('Ctrl Pts',(16.6476240631459,-0.436436950410268,
11.4038283027745));
#22436=CARTESIAN_POINT('Ctrl Pts',(16.0510567137341,-0.751891803416538,
-3.01914151387231));
#22437=CARTESIAN_POINT('Ctrl Pts',(16.0510567137341,-0.751891803416538,
11.4038283027745));
#22438=CARTESIAN_POINT('Ctrl Pts',(15.6027736445726,-1.21202503656501,-3.01914151387231));
#22439=CARTESIAN_POINT('Ctrl Pts',(15.6027736445726,-1.21202503656501,11.4038283027745));
#22440=CARTESIAN_POINT('Ctrl Pts',(15.2713584598603,-1.58690028117533,-3.01914151387231));
#22441=CARTESIAN_POINT('Ctrl Pts',(15.2713584598603,-1.58690028117533,11.4038283027745));
#22442=CARTESIAN_POINT('Ctrl Pts',(14.8456161221497,-2.0684722499697,-3.01914151387231));
#22443=CARTESIAN_POINT('Ctrl Pts',(14.8456161221497,-2.0684722499697,11.4038283027745));
#22444=CARTESIAN_POINT('Ctrl Pts',(14.5613685394243,-2.40143629916816,-3.01914151387231));
#22445=CARTESIAN_POINT('Ctrl Pts',(14.5613685394243,-2.40143629916816,11.4038283027745));
#22446=CARTESIAN_POINT('Ctrl Pts',(14.3828812435025,-2.53302458721095,-3.01914151387231));
#22447=CARTESIAN_POINT('Ctrl Pts',(14.3828812435025,-2.53302458721095,11.4038283027745));
#22448=CARTESIAN_POINT('Ctrl Pts',(14.201535511025,-2.66672023404866,-3.01914151387231));
#22449=CARTESIAN_POINT('Ctrl Pts',(14.201535511025,-2.66672023404866,11.4038283027745));
#22450=CARTESIAN_POINT('Ctrl Pts',(14.14690312219,-2.68051922028271,-3.01914151387231));
#22451=CARTESIAN_POINT('Ctrl Pts',(14.14690312219,-2.68051922028271,11.4038283027745));
#22452=CARTESIAN_POINT('Ctrl Pts',(13.9521549326808,-2.68051922028271,-3.01914151387231));
#22453=CARTESIAN_POINT('Ctrl Pts',(13.9521549326808,-2.68051922028271,11.4038283027745));
#22454=CARTESIAN_POINT('',(13.9521549326808,-2.68051922028271,-0.737782898536615));
#22455=CARTESIAN_POINT('Ctrl Pts',(18.2877536206758,3.39996748803095E-6,
-0.737782898536615));
#22456=CARTESIAN_POINT('Ctrl Pts',(18.2831008061387,-0.000306707045958711,
-0.737782898536615));
#22457=CARTESIAN_POINT('Ctrl Pts',(18.278434780269,-0.000621741973328828,
-0.737782898536615));
#22458=CARTESIAN_POINT('Ctrl Pts',(17.815024722384,-0.0323158724884442,
-0.737782898536615));
#22459=CARTESIAN_POINT('Ctrl Pts',(17.2029954141084,-0.14276585350144,-0.737782898536615));
#22460=CARTESIAN_POINT('Ctrl Pts',(16.0510567137341,-0.751891803416538,
-0.737782898536615));
#22461=CARTESIAN_POINT('Ctrl Pts',(15.6027736445726,-1.21202503656501,-0.737782898536615));
#22462=CARTESIAN_POINT('Ctrl Pts',(14.8456161221497,-2.0684722499697,-0.737782898536615));
#22463=CARTESIAN_POINT('Ctrl Pts',(14.5613685394243,-2.40143629916816,-0.737782898536615));
#22464=CARTESIAN_POINT('Ctrl Pts',(14.201535511025,-2.66672023404866,-0.737782898536615));
#22465=CARTESIAN_POINT('Ctrl Pts',(14.14690312219,-2.68051922028271,-0.737782898536615));
#22466=CARTESIAN_POINT('Ctrl Pts',(13.9521549326808,-2.68051922028271,-0.737782898536615));
#22467=CARTESIAN_POINT('',(13.9521549326808,-2.68051922028271,5.59936274946018));
#22468=CARTESIAN_POINT('',(13.9521549326808,-2.68051922028271,0.));
#22469=CARTESIAN_POINT('Ctrl Pts',(13.9521549326808,-2.68051922028271,5.59936274946018));
#22470=CARTESIAN_POINT('Ctrl Pts',(14.14690312219,-2.68051922028271,5.59936274946018));
#22471=CARTESIAN_POINT('Ctrl Pts',(14.201535511025,-2.66672023404866,5.59936274946018));
#22472=CARTESIAN_POINT('Ctrl Pts',(14.3828812435025,-2.53302458721095,5.59936274946018));
#22473=CARTESIAN_POINT('Ctrl Pts',(14.5613685394243,-2.40143629916816,5.59936274946018));
#22474=CARTESIAN_POINT('Ctrl Pts',(14.8456161221497,-2.0684722499697,5.59936274946018));
#22475=CARTESIAN_POINT('Ctrl Pts',(15.2713584598603,-1.58690028117533,5.59936274946018));
#22476=CARTESIAN_POINT('Ctrl Pts',(15.6027736445726,-1.21202503656501,5.59936274946018));
#22477=CARTESIAN_POINT('Ctrl Pts',(16.0510567137341,-0.751891803416538,
5.59936274946018));
#22478=CARTESIAN_POINT('Ctrl Pts',(16.6476240631459,-0.436436950410268,
5.59936274946018));
#22479=CARTESIAN_POINT('Ctrl Pts',(17.2029954141084,-0.14276585350144,5.59936274946018));
#22480=CARTESIAN_POINT('Ctrl Pts',(17.815024722384,-0.0323158724884442,
5.59936274946018));
#22481=CARTESIAN_POINT('Ctrl Pts',(18.2737554003772,-0.00094178007888357,
5.59936274946018));
#22482=CARTESIAN_POINT('Ctrl Pts',(18.2784351727308,-0.000621715131582311,
5.59936274946018));
#22483=CARTESIAN_POINT('Ctrl Pts',(18.2831015888222,-0.000306654201738675,
5.59936274946018));
#22484=CARTESIAN_POINT('Ctrl Pts',(18.2877547913768,3.477993847498E-6,5.59936274946018));
#22485=CARTESIAN_POINT('Origin',(-1.89430524244949,0.,-0.737782898536615));
#22486=CARTESIAN_POINT('',(20.1650770882888,-1.63165946910082,-0.737782898536615));
#22487=CARTESIAN_POINT('',(20.1650770882888,0.,-0.737782898536615));
#22488=CARTESIAN_POINT('',(19.2071026744088,-1.63165946910082,-0.737782898536615));
#22489=CARTESIAN_POINT('',(8.65639871597966,-1.63165946910082,-0.737782898536615));
#22490=CARTESIAN_POINT('',(13.9521549326808,-4.33051922028271,-0.737782898536615));
#22491=CARTESIAN_POINT('Ctrl Pts',(13.9521549326808,-4.33051922028271,-0.737782898536615));
#22492=CARTESIAN_POINT('Ctrl Pts',(14.0367700658778,-4.33051922028271,-0.737782898536615));
#22493=CARTESIAN_POINT('Ctrl Pts',(14.2036369078635,-4.3237071977066,-0.737782898536615));
#22494=CARTESIAN_POINT('Ctrl Pts',(14.4468469322399,-4.29305314840303,-0.737782898536615));
#22495=CARTESIAN_POINT('Ctrl Pts',(14.7569409494257,-4.21100033264776,-0.737782898536615));
#22496=CARTESIAN_POINT('Ctrl Pts',(15.1212896693278,-4.03949049111154,-0.737782898536615));
#22497=CARTESIAN_POINT('Ctrl Pts',(15.4636185066764,-3.80138932605477,-0.737782898536615));
#22498=CARTESIAN_POINT('Ctrl Pts',(15.7866049591328,-3.50410652905647,-0.737782898536615));
#22499=CARTESIAN_POINT('Ctrl Pts',(16.0950135392462,-3.16285055044176,-0.737782898536615));
#22500=CARTESIAN_POINT('Ctrl Pts',(16.396392567999,-2.80347808583323,-0.737782898536615));
#22501=CARTESIAN_POINT('Ctrl Pts',(16.6994685020962,-2.45665970286042,-0.737782898536615));
#22502=CARTESIAN_POINT('Ctrl Pts',(17.0126841408516,-2.15256650575318,-0.737782898536615));
#22503=CARTESIAN_POINT('Ctrl Pts',(17.3426063821155,-1.91508101584403,-0.737782898536615));
#22504=CARTESIAN_POINT('Ctrl Pts',(17.6925082784732,-1.75662630260534,-0.737782898536615));
#22505=CARTESIAN_POINT('Ctrl Pts',(18.0602469444161,-1.6704655276535,-0.737782898536615));
#22506=CARTESIAN_POINT('Ctrl Pts',(18.4399535686149,-1.63662374391445,-0.737782898536615));
#22507=CARTESIAN_POINT('Ctrl Pts',(18.7476534820197,-1.63200385678456,-0.737782898536615));
#22508=CARTESIAN_POINT('Ctrl Pts',(18.9779068684107,-1.63172180635354,-0.737782898536615));
#22509=CARTESIAN_POINT('Ctrl Pts',(19.1308048362197,-1.63165946910082,-0.737782898536615));
#22510=CARTESIAN_POINT('Ctrl Pts',(19.2071026744088,-1.63165946910082,-0.737782898536615));
#22511=CARTESIAN_POINT('',(5.09382715545311,-4.33051922028271,-0.737782898536615));
#22512=CARTESIAN_POINT('',(1.59976095650181,-4.33051922028271,-0.737782898536615));
#22513=CARTESIAN_POINT('Origin',(5.09382715545311,0.,-0.737782898536615));
#22514=CARTESIAN_POINT('',(5.1457717363639,-2.6650130345292,-0.737782898536615));
#22515=CARTESIAN_POINT('Origin',(5.09382715545311,0.,-0.737782898536615));
#22516=CARTESIAN_POINT('',(5.1457717363639,-2.68051922028271,-0.737782898536615));
#22517=CARTESIAN_POINT('',(5.1457717363639,-1.34025961014136,-0.737782898536615));
#22518=CARTESIAN_POINT('',(6.02892484511565,-2.68051922028271,-0.737782898536615));
#22519=CARTESIAN_POINT('Ctrl Pts',(20.1650770882888,-12.,-0.737782898536615));
#22520=CARTESIAN_POINT('Ctrl Pts',(20.1650770882888,16.8,-0.737782898536615));
#22521=CARTESIAN_POINT('Ctrl Pts',(20.2051790492699,-12.,-0.737782898536615));
#22522=CARTESIAN_POINT('Ctrl Pts',(20.2051790492699,16.8,-0.737782898536615));
#22523=CARTESIAN_POINT('Ctrl Pts',(20.2856318058959,-12.,-0.738334262610078));
#22524=CARTESIAN_POINT('Ctrl Pts',(20.2856318058959,16.8,-0.738334262610078));
#22525=CARTESIAN_POINT('Ctrl Pts',(20.4070574409421,-12.,-0.740817279017836));
#22526=CARTESIAN_POINT('Ctrl Pts',(20.4070574409421,16.8,-0.740817279017836));
#22527=CARTESIAN_POINT('Ctrl Pts',(20.570466834294,-12.,-0.750031355028731));
#22528=CARTESIAN_POINT('Ctrl Pts',(20.570466834294,16.8,-0.750031355028731));
#22529=CARTESIAN_POINT('Ctrl Pts',(20.7773607278973,-12.,-0.785302229564316));
#22530=CARTESIAN_POINT('Ctrl Pts',(20.7773607278973,16.8,-0.785302229564316));
#22531=CARTESIAN_POINT('Ctrl Pts',(20.9870805449298,-12.,-0.859882777793607));
#22532=CARTESIAN_POINT('Ctrl Pts',(20.9870805449298,16.8,-0.859882777793607));
#22533=CARTESIAN_POINT('Ctrl Pts',(21.1998878964781,-12.,-0.985918438087056));
#22534=CARTESIAN_POINT('Ctrl Pts',(21.1998878964781,16.8,-0.985918438087056));
#22535=CARTESIAN_POINT('Ctrl Pts',(21.4160984502468,-12.,-1.16513193018819));
#22536=CARTESIAN_POINT('Ctrl Pts',(21.4160984502468,16.8,-1.16513193018819));
#22537=CARTESIAN_POINT('Ctrl Pts',(21.6360629244597,-12.,-1.38851558520595));
#22538=CARTESIAN_POINT('Ctrl Pts',(21.6360629244597,16.8,-1.38851558520595));
#22539=CARTESIAN_POINT('Ctrl Pts',(21.8601428560791,-12.,-1.64103427806176));
#22540=CARTESIAN_POINT('Ctrl Pts',(21.8601428560791,16.8,-1.64103427806176));
#22541=CARTESIAN_POINT('Ctrl Pts',(22.0886743686473,-12.,-1.90460559759654));
#22542=CARTESIAN_POINT('Ctrl Pts',(22.0886743686473,16.8,-1.90460559759654));
#22543=CARTESIAN_POINT('Ctrl Pts',(22.3219273279567,-12.,-2.16140314464429));
#22544=CARTESIAN_POINT('Ctrl Pts',(22.3219273279567,16.8,-2.16140314464429));
#22545=CARTESIAN_POINT('Ctrl Pts',(22.5600378010161,-12.,-2.3973000769867));
#22546=CARTESIAN_POINT('Ctrl Pts',(22.5600378010161,16.8,-2.3973000769867));
#22547=CARTESIAN_POINT('Ctrl Pts',(22.8029682104327,-12.,-2.60422537589526));
#22548=CARTESIAN_POINT('Ctrl Pts',(22.8029682104327,16.8,-2.60422537589526));
#22549=CARTESIAN_POINT('Ctrl Pts',(23.0506005766976,-12.,-2.77805908652226));
#22550=CARTESIAN_POINT('Ctrl Pts',(23.0506005766976,16.8,-2.77805908652226));
#22551=CARTESIAN_POINT('Ctrl Pts',(23.2523538070279,-12.,-2.88956861747599));
#22552=CARTESIAN_POINT('Ctrl Pts',(23.2523538070279,16.8,-2.88956861747599));
#22553=CARTESIAN_POINT('Ctrl Pts',(23.4056687844597,-12.,-2.95772702235629));
#22554=CARTESIAN_POINT('Ctrl Pts',(23.4056687844597,16.8,-2.95772702235629));
#22555=CARTESIAN_POINT('Ctrl Pts',(23.5087612184661,-12.,-2.99633939947042));
#22556=CARTESIAN_POINT('Ctrl Pts',(23.5087612184661,16.8,-2.99633939947042));
#22557=CARTESIAN_POINT('Ctrl Pts',(23.560528050594,-12.,-3.01393888949139));
#22558=CARTESIAN_POINT('Ctrl Pts',(23.560528050594,16.8,-3.01393888949139));
#22559=CARTESIAN_POINT('',(23.5207683417462,-1.63165946910082,-3.));
#22560=CARTESIAN_POINT('',(23.5207683417462,-1.63165946910082,-3.));
#22561=CARTESIAN_POINT('Ctrl Pts',(20.1650770882888,-1.63165946910082,-0.737782898536615));
#22562=CARTESIAN_POINT('Ctrl Pts',(20.2051790492699,-1.63165946910082,-0.737782898536615));
#22563=CARTESIAN_POINT('Ctrl Pts',(20.2856318058959,-1.63165946910082,-0.738334262610078));
#22564=CARTESIAN_POINT('Ctrl Pts',(20.4070574409421,-1.63165946910082,-0.740817279017836));
#22565=CARTESIAN_POINT('Ctrl Pts',(20.570466834294,-1.63165946910082,-0.750031355028731));
#22566=CARTESIAN_POINT('Ctrl Pts',(20.7773607278973,-1.63165946910082,-0.785302229564316));
#22567=CARTESIAN_POINT('Ctrl Pts',(20.9870805449298,-1.63165946910082,-0.859882777793607));
#22568=CARTESIAN_POINT('Ctrl Pts',(21.1998878964781,-1.63165946910082,-0.985918438087056));
#22569=CARTESIAN_POINT('Ctrl Pts',(21.4160984502468,-1.63165946910082,-1.16513193018819));
#22570=CARTESIAN_POINT('Ctrl Pts',(21.6360629244597,-1.63165946910082,-1.38851558520595));
#22571=CARTESIAN_POINT('Ctrl Pts',(21.8601428560791,-1.63165946910082,-1.64103427806176));
#22572=CARTESIAN_POINT('Ctrl Pts',(22.0886743686473,-1.63165946910082,-1.90460559759654));
#22573=CARTESIAN_POINT('Ctrl Pts',(22.3219273279567,-1.63165946910082,-2.16140314464429));
#22574=CARTESIAN_POINT('Ctrl Pts',(22.5600378010161,-1.63165946910082,-2.3973000769867));
#22575=CARTESIAN_POINT('Ctrl Pts',(22.8029682104327,-1.63165946910082,-2.60422537589526));
#22576=CARTESIAN_POINT('Ctrl Pts',(23.0429827907474,-1.63165946910082,-2.77271153031038));
#22577=CARTESIAN_POINT('Ctrl Pts',(23.2368431253681,-1.63165946910082,-2.88095209536456));
#22578=CARTESIAN_POINT('Ctrl Pts',(23.3821028186481,-1.63165946910082,-2.94712138325619));
#22579=CARTESIAN_POINT('Ctrl Pts',(23.4770787559704,-1.63165946910082,-2.98421892689512));
#22580=CARTESIAN_POINT('Ctrl Pts',(23.5207683417462,-1.63165946910082,-3.));
#22581=CARTESIAN_POINT('Origin',(14.1696121318917,-2.14824178200142,-3.));
#22582=CARTESIAN_POINT('',(25.8992960798277,-1.63165946910082,-3.));
#22583=CARTESIAN_POINT('',(25.8992960798277,0.,-3.));
#22584=CARTESIAN_POINT('',(19.2071026744088,-1.63165946910082,-3.));
#22585=CARTESIAN_POINT('Origin',(24.7143466872546,0.,-0.395297377936459));
#22586=CARTESIAN_POINT('',(27.575916328613,-1.63165946910082,-0.395297377936459));
#22587=CARTESIAN_POINT('',(27.575916328613,0.,-0.395297377936459));
#22588=CARTESIAN_POINT('Origin',(24.7143466872546,-1.63165946910082,-0.395297377936459));
#22589=CARTESIAN_POINT('Origin',(24.7143466872546,0.,5.90470262206354));
#22590=CARTESIAN_POINT('',(21.9988718582129,-1.63165946910082,6.80735275649273));
#22591=CARTESIAN_POINT('',(21.9988718582129,0.,6.80735275649273));
#22592=CARTESIAN_POINT('',(27.575916328613,-1.63165946910082,5.90470262206354));
#22593=CARTESIAN_POINT('Origin',(24.7143466872546,-1.63165946910082,5.90470262206354));
#22594=CARTESIAN_POINT('',(27.575916328613,0.,5.90470262206354));
#22595=CARTESIAN_POINT('Origin',(20.1650770882888,0.,7.59525803303831));
#22596=CARTESIAN_POINT('',(20.1650770882888,-1.63165946910082,5.59936274946018));
#22597=CARTESIAN_POINT('',(20.1650770882888,0.,5.59936274946018));
#22598=CARTESIAN_POINT('Origin',(20.1650770882888,-1.63165946910082,7.59525803303831));
#22599=CARTESIAN_POINT('Origin',(20.1650770882888,0.,5.59936274946018));
#22600=CARTESIAN_POINT('',(5.09382715545311,-4.33051922028271,5.59936274946018));
#22601=CARTESIAN_POINT('Origin',(5.09382715545311,0.,5.59936274946018));
#22602=CARTESIAN_POINT('',(13.9521549326808,-4.33051922028271,5.59936274946018));
#22603=CARTESIAN_POINT('',(12.629452121871,-4.33051922028271,5.59936274946018));
#22604=CARTESIAN_POINT('',(19.2071026744088,-1.63165946910082,5.59936274946018));
#22605=CARTESIAN_POINT('Ctrl Pts',(19.2071026744088,-1.63165946910082,5.59936274946018));
#22606=CARTESIAN_POINT('Ctrl Pts',(19.1308048362197,-1.63165946910082,5.59936274946018));
#22607=CARTESIAN_POINT('Ctrl Pts',(18.9779068684107,-1.63172180635354,5.59936274946018));
#22608=CARTESIAN_POINT('Ctrl Pts',(18.7476534820197,-1.63200385678456,5.59936274946018));
#22609=CARTESIAN_POINT('Ctrl Pts',(18.4399535686149,-1.63662374391445,5.59936274946018));
#22610=CARTESIAN_POINT('Ctrl Pts',(18.0602469444161,-1.6704655276535,5.59936274946018));
#22611=CARTESIAN_POINT('Ctrl Pts',(17.6925082784732,-1.75662630260534,5.59936274946018));
#22612=CARTESIAN_POINT('Ctrl Pts',(17.3426063821155,-1.91508101584403,5.59936274946018));
#22613=CARTESIAN_POINT('Ctrl Pts',(17.0126841408516,-2.15256650575318,5.59936274946018));
#22614=CARTESIAN_POINT('Ctrl Pts',(16.6994685020962,-2.45665970286042,5.59936274946018));
#22615=CARTESIAN_POINT('Ctrl Pts',(16.396392567999,-2.80347808583323,5.59936274946018));
#22616=CARTESIAN_POINT('Ctrl Pts',(16.0950135392462,-3.16285055044176,5.59936274946018));
#22617=CARTESIAN_POINT('Ctrl Pts',(15.7866049591328,-3.50410652905647,5.59936274946018));
#22618=CARTESIAN_POINT('Ctrl Pts',(15.4636185066764,-3.80138932605477,5.59936274946018));
#22619=CARTESIAN_POINT('Ctrl Pts',(15.1212896693278,-4.03949049111154,5.59936274946018));
#22620=CARTESIAN_POINT('Ctrl Pts',(14.7569409494257,-4.21100033264776,5.59936274946018));
#22621=CARTESIAN_POINT('Ctrl Pts',(14.4468469322399,-4.29305314840303,5.59936274946018));
#22622=CARTESIAN_POINT('Ctrl Pts',(14.2036369078635,-4.3237071977066,5.59936274946018));
#22623=CARTESIAN_POINT('Ctrl Pts',(14.0367700658778,-4.33051922028271,5.59936274946018));
#22624=CARTESIAN_POINT('Ctrl Pts',(13.9521549326808,-4.33051922028271,5.59936274946018));
#22625=CARTESIAN_POINT('',(19.6860898813488,-1.63165946910082,5.59936274946018));
#22626=CARTESIAN_POINT('',(5.1457717363639,-2.68051922028271,5.59936274946018));
#22627=CARTESIAN_POINT('',(17.0586160104848,-2.68051922028271,5.59936274946018));
#22628=CARTESIAN_POINT('',(5.1457717363639,-2.6650130345292,5.59936274946018));
#22629=CARTESIAN_POINT('',(5.1457717363639,-1.34025961014136,5.59936274946018));
#22630=CARTESIAN_POINT('Origin',(5.09382715545311,0.,5.59936274946018));
#22631=CARTESIAN_POINT('Origin',(24.7143466872546,0.,5.90470262206354));
#22632=CARTESIAN_POINT('',(23.013011518287,-1.63165946910082,5.90470262206354));
#22633=CARTESIAN_POINT('Origin',(24.7143466872546,-1.63165946910082,5.90470262206354));
#22634=CARTESIAN_POINT('',(23.013011518287,0.,5.90470262206354));
#22635=CARTESIAN_POINT('Origin',(24.7143466872546,0.,-0.395297377936459));
#22636=CARTESIAN_POINT('',(23.013011518287,-1.63165946910082,-0.395297377936459));
#22637=CARTESIAN_POINT('Origin',(24.7143466872546,-1.63165946910082,-0.395297377936459));
#22638=CARTESIAN_POINT('',(23.013011518287,0.,-0.395297377936459));
#22639=CARTESIAN_POINT('Origin',(27.575916328613,-1.63165946910082,0.));
#22640=CARTESIAN_POINT('',(27.575916328613,-1.63165946910082,0.));
#22641=CARTESIAN_POINT('Ctrl Pts',(13.9521549326808,-4.33051922028271,-3.));
#22642=CARTESIAN_POINT('Ctrl Pts',(13.9521549326808,-4.33051922028271,11.4));
#22643=CARTESIAN_POINT('Ctrl Pts',(14.0367700658778,-4.33051922028271,-3.));
#22644=CARTESIAN_POINT('Ctrl Pts',(14.0367700658778,-4.33051922028271,11.4));
#22645=CARTESIAN_POINT('Ctrl Pts',(14.2036369078635,-4.3237071977066,-3.));
#22646=CARTESIAN_POINT('Ctrl Pts',(14.2036369078635,-4.3237071977066,11.4));
#22647=CARTESIAN_POINT('Ctrl Pts',(14.4468469322399,-4.29305314840303,-3.));
#22648=CARTESIAN_POINT('Ctrl Pts',(14.4468469322399,-4.29305314840303,11.4));
#22649=CARTESIAN_POINT('Ctrl Pts',(14.7569409494257,-4.21100033264776,-3.));
#22650=CARTESIAN_POINT('Ctrl Pts',(14.7569409494257,-4.21100033264776,11.4));
#22651=CARTESIAN_POINT('Ctrl Pts',(15.1212896693278,-4.03949049111154,-3.));
#22652=CARTESIAN_POINT('Ctrl Pts',(15.1212896693278,-4.03949049111154,11.4));
#22653=CARTESIAN_POINT('Ctrl Pts',(15.4636185066764,-3.80138932605477,-3.));
#22654=CARTESIAN_POINT('Ctrl Pts',(15.4636185066764,-3.80138932605477,11.4));
#22655=CARTESIAN_POINT('Ctrl Pts',(15.7866049591328,-3.50410652905647,-3.));
#22656=CARTESIAN_POINT('Ctrl Pts',(15.7866049591328,-3.50410652905647,11.4));
#22657=CARTESIAN_POINT('Ctrl Pts',(16.0950135392462,-3.16285055044176,-3.));
#22658=CARTESIAN_POINT('Ctrl Pts',(16.0950135392462,-3.16285055044176,11.4));
#22659=CARTESIAN_POINT('Ctrl Pts',(16.396392567999,-2.80347808583323,-3.));
#22660=CARTESIAN_POINT('Ctrl Pts',(16.396392567999,-2.80347808583323,11.4));
#22661=CARTESIAN_POINT('Ctrl Pts',(16.6994685020962,-2.45665970286042,-3.));
#22662=CARTESIAN_POINT('Ctrl Pts',(16.6994685020962,-2.45665970286042,11.4));
#22663=CARTESIAN_POINT('Ctrl Pts',(17.0126841408516,-2.15256650575318,-3.));
#22664=CARTESIAN_POINT('Ctrl Pts',(17.0126841408516,-2.15256650575318,11.4));
#22665=CARTESIAN_POINT('Ctrl Pts',(17.3426063821155,-1.91508101584403,-3.));
#22666=CARTESIAN_POINT('Ctrl Pts',(17.3426063821155,-1.91508101584403,11.4));
#22667=CARTESIAN_POINT('Ctrl Pts',(17.6925082784732,-1.75662630260534,-3.));
#22668=CARTESIAN_POINT('Ctrl Pts',(17.6925082784732,-1.75662630260534,11.4));
#22669=CARTESIAN_POINT('Ctrl Pts',(18.0602469444161,-1.6704655276535,-3.));
#22670=CARTESIAN_POINT('Ctrl Pts',(18.0602469444161,-1.6704655276535,11.4));
#22671=CARTESIAN_POINT('Ctrl Pts',(18.4399535686149,-1.63662374391445,-3.));
#22672=CARTESIAN_POINT('Ctrl Pts',(18.4399535686149,-1.63662374391445,11.4));
#22673=CARTESIAN_POINT('Ctrl Pts',(18.7476534820197,-1.63200385678456,-3.));
#22674=CARTESIAN_POINT('Ctrl Pts',(18.7476534820197,-1.63200385678456,11.4));
#22675=CARTESIAN_POINT('Ctrl Pts',(18.9779068684107,-1.63172180635354,-3.));
#22676=CARTESIAN_POINT('Ctrl Pts',(18.9779068684107,-1.63172180635354,11.4));
#22677=CARTESIAN_POINT('Ctrl Pts',(19.1308048362197,-1.63165946910082,-3.));
#22678=CARTESIAN_POINT('Ctrl Pts',(19.1308048362197,-1.63165946910082,11.4));
#22679=CARTESIAN_POINT('Ctrl Pts',(19.2071026744088,-1.63165946910082,-3.));
#22680=CARTESIAN_POINT('Ctrl Pts',(19.2071026744088,-1.63165946910082,11.4));
#22681=CARTESIAN_POINT('',(19.2071026744088,-1.63165946910082,0.));
#22682=CARTESIAN_POINT('',(13.9521549326808,-4.33051922028271,0.));
#22683=CARTESIAN_POINT('Origin',(19.2071026744088,-1.63165946910082,0.));
#22684=CARTESIAN_POINT('Origin',(5.09382715545311,-4.33051922028271,0.));
#22685=CARTESIAN_POINT('',(5.09382715545311,-4.33051922028271,0.));
#22686=CARTESIAN_POINT('Origin',(5.09382715545311,0.,0.));
#22687=CARTESIAN_POINT('Origin',(5.09382715545311,0.,0.));
#22688=CARTESIAN_POINT('',(5.1457717363639,-2.6650130345292,0.));
#22689=CARTESIAN_POINT('Origin',(5.1457717363639,-2.68051922028271,0.));
#22690=CARTESIAN_POINT('',(5.1457717363639,-2.68051922028271,0.));
#22691=CARTESIAN_POINT('Origin',(13.9521549326808,-2.68051922028271,0.));
#23564=UNCERTAINTY_MEASURE_WITH_UNIT(LENGTH_MEASURE(0.01),#23578,
'DISTANCE_ACCURACY_VALUE',
'Maximum model space distance between geometric entities at asserted c
onnectivities');
#23566=UNCERTAINTY_MEASURE_WITH_UNIT(LENGTH_MEASURE(0.01),#23578,
'DISTANCE_ACCURACY_VALUE',
'Maximum model space distance between geometric entities at asserted c
onnectivities');
#23575=(
GEOMETRIC_REPRESENTATION_CONTEXT(3)
GLOBAL_UNCERTAINTY_ASSIGNED_CONTEXT((#23564))
GLOBAL_UNIT_ASSIGNED_CONTEXT((#23578,#23580,#23581))
REPRESENTATION_CONTEXT('','3D')
);
#23577=(
GEOMETRIC_REPRESENTATION_CONTEXT(3)
GLOBAL_UNCERTAINTY_ASSIGNED_CONTEXT((#23566))
GLOBAL_UNIT_ASSIGNED_CONTEXT((#23578,#23580,#23581))
REPRESENTATION_CONTEXT('','3D')
);
#23578=(
LENGTH_UNIT()
NAMED_UNIT(*)
SI_UNIT(.MILLI.,.METRE.)
);
#23580=(
NAMED_UNIT(*)
PLANE_ANGLE_UNIT()
SI_UNIT($,.RADIAN.)
);
#23581=(
NAMED_UNIT(*)
SI_UNIT($,.STERADIAN.)
SOLID_ANGLE_UNIT()
);
#23590=SHAPE_DEFINITION_REPRESENTATION(#23600,#23619);
#23600=PRODUCT_DEFINITION_SHAPE('',$,#23630);
#23619=SHAPE_REPRESENTATION('',(#4573),#23575);
#23621=PRODUCT_DEFINITION_CONTEXT('part definition',#23653,'design');
#23630=PRODUCT_DEFINITION('Clamp_02','Clamp_02',#23640,#23621);
#23640=PRODUCT_DEFINITION_FORMATION('',$,#23663);
#23653=APPLICATION_CONTEXT(
'Core Data for Automotive Mechanical Design Process');
#23654=PRODUCT_CONTEXT('part definition',#23653,'mechanical');
#23663=PRODUCT('Clamp_02','Clamp_02',$,(#23654));
#23666=PRESENTATION_STYLE_ASSIGNMENT((#23671));
#23671=SURFACE_STYLE_USAGE(.BOTH.,#23676);
#23676=SURFACE_SIDE_STYLE('',(#23681));
#23681=SURFACE_STYLE_FILL_AREA(#23686);
#23686=FILL_AREA_STYLE('Opaque(210,210,210)',(#23691));
#23691=FILL_AREA_STYLE_COLOUR('Opaque(210,210,210)',#23696);
#23696=COLOUR_RGB('Opaque(210,210,210)', 0.09019608, 0.27058824, 0.51372549);
ENDSEC;
END-ISO-10303-21;
